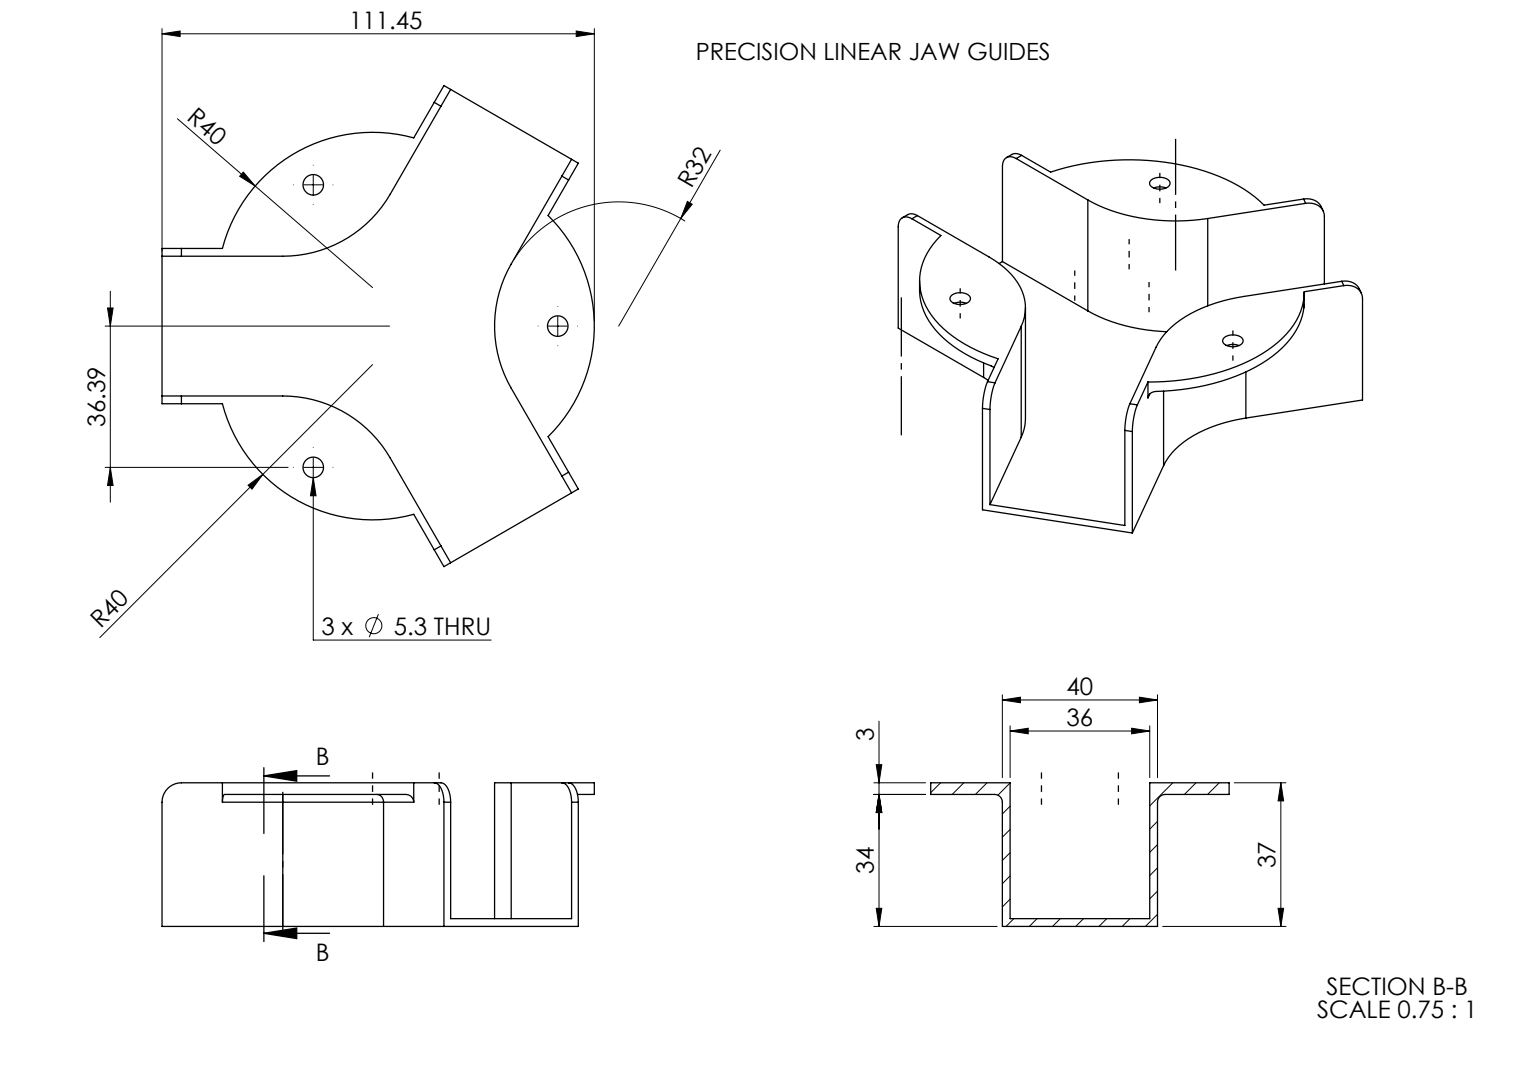
ISO-10303-21;
HEADER;
FILE_DESCRIPTION (('STEP AP214'),
    '1' );
FILE_NAME ('Precision Linear Jaw Guides.step',
    '2026-10-08T13:56:24',
    ( '' ),
    ( '' ),
    'SwSTEP 2.0',
    'SolidWorks 2026',
    '' );
FILE_SCHEMA (( 'AUTOMOTIVE_DESIGN' ));
ENDSEC;

DATA;
#1=ORIENTED_EDGE ( 'NONE', *, *, #6878, .F. ) ;
#24=ORIENTED_EDGE ( 'NONE', *, *, #9310, .F. ) ;
#44=CARTESIAN_POINT ( 'NONE',  ( 45.58845726811988897, -5.000000000000004441, 42.96152422706634155 ) ) ;
#63=EDGE_CURVE ( 'NONE', #10036, #14429, #10056, .T. ) ;
#65=CARTESIAN_POINT ( 'NONE',  ( 4.896370289181515290, -5.000000000000000000, 48.48076211353313170 ) ) ;
#73=FACE_OUTER_BOUND ( 'NONE', #11557, .T. ) ;
#75=ORIENTED_EDGE ( 'NONE', *, *, #13958, .T. ) ;
#102=EDGE_CURVE ( 'NONE', #3403, #4061, #7930, .T. ) ;
#103=CARTESIAN_POINT ( 'NONE',  ( 40.98096197216263903, -3.000000000000000000, 26.98110827883376928 ) ) ;
#118=DIRECTION ( 'NONE',  ( 0.000000000000000000, 0.000000000000000000, -1.000000000000000000 ) ) ;
#135=EDGE_LOOP ( 'NONE', ( #5012, #11685, #4576, #2768 ) ) ;
#159=ORIENTED_EDGE ( 'NONE', *, *, #7096, .F. ) ;
#161=CARTESIAN_POINT ( 'NONE',  ( 11.91154273188013768, 0.000000000000000000, -56.63139720814412925 ) ) ;
#162=AXIS2_PLACEMENT_3D ( 'NONE', #1282, #2402, #6227 ) ;
#178=PRESENTATION_STYLE_ASSIGNMENT (( #1292 ) ) ;
#181=ORIENTED_EDGE ( 'NONE', *, *, #2624, .T. ) ;
#183=EDGE_CURVE ( 'NONE', #10747, #715, #1391, .T. ) ;
#184=ORIENTED_EDGE ( 'NONE', *, *, #8002, .F. ) ;
#191=CARTESIAN_POINT ( 'NONE',  ( 39.53738644055469820, -5.000000000000000000, -28.48076211352550047 ) ) ;
#200=( NAMED_UNIT ( * ) SI_UNIT ( $, .STERADIAN. ) SOLID_ANGLE_UNIT ( ) );
#201=ORIENTED_EDGE ( 'NONE', *, *, #2412, .F. ) ;
#202=FACE_OUTER_BOUND ( 'NONE', #2206, .T. ) ;
#205=EDGE_CURVE ( 'NONE', #14772, #10685, #7688, .T. ) ;
#213=AXIS2_PLACEMENT_3D ( 'NONE', #6440, #11355, #304 ) ;
#233=VECTOR ( 'NONE', #8677, 1000.000000000000114 ) ;
#254=ORIENTED_EDGE ( 'NONE', *, *, #15050, .F. ) ;
#275=EDGE_CURVE ( 'NONE', #7055, #3403, #5959, .T. ) ;
#285=ORIENTED_EDGE ( 'NONE', *, *, #7627, .F. ) ;
#287=CARTESIAN_POINT ( 'NONE',  ( -28.86751345948129455, -35.00000000000000000, 49.99999999999999289 ) ) ;
#304=DIRECTION ( 'NONE',  ( 0.000000000000000000, 0.000000000000000000, 1.000000000000000000 ) ) ;
#342=FILL_AREA_STYLE ('',( #5011 ) ) ;
#347=AXIS2_PLACEMENT_3D ( 'NONE', #11601, #15335, #628 ) ;
#359=ORIENTED_EDGE ( 'NONE', *, *, #11812, .F. ) ;
#362=VERTEX_POINT ( 'NONE', #11512 ) ;
#381=ADVANCED_FACE ( 'NONE', ( #13861 ), #3996, .T. ) ;
#388=PLANE ( 'NONE',  #14679 ) ;
#395=VERTEX_POINT ( 'NONE', #15166 ) ;
#421=CARTESIAN_POINT ( 'NONE',  ( -44.05158835363087633, -3.098194602941751530, 21.36784885013319624 ) ) ;
#425=DIRECTION ( 'NONE',  ( -1.000000000000000000, 0.000000000000000000, 0.000000000000000000 ) ) ;
#435=LINE ( 'NONE', #9087, #7748 ) ;
#441=CIRCLE ( 'NONE', #4826, 29.99999999999999289 ) ;
#465=DIRECTION ( 'NONE',  ( 8.673617379884034486E-16, 0.000000000000000000, 1.000000000000000000 ) ) ;
#475=EDGE_CURVE ( 'NONE', #1675, #4627, #623, .T. ) ;
#478=EDGE_LOOP ( 'NONE', ( #2495, #13300, #2111, #13302 ) ) ;
#482=VERTEX_POINT ( 'NONE', #13120 ) ;
#487=ORIENTED_EDGE ( 'NONE', *, *, #7096, .T. ) ;
#492=AXIS2_PLACEMENT_3D ( 'NONE', #7401, #13083, #5207 ) ;
#512=VECTOR ( 'NONE', #11630, 1000.000000000000000 ) ;
#516=CARTESIAN_POINT ( 'NONE',  ( 47.32050807568879947, -37.00000000000000711, -41.96152422706630603 ) ) ;
#519=ADVANCED_FACE ( 'NONE', ( #932 ), #7080, .T. ) ;
#526=EDGE_LOOP ( 'NONE', ( #2721, #11527, #12496, #1351, #6317, #10390, #12512 ) ) ;
#534=EDGE_CURVE ( 'NONE', #9400, #9517, #9860, .T. ) ;
#536=DIRECTION ( 'NONE',  ( -0.8660254037844388186, -0.000000000000000000, 0.4999999999999998890 ) ) ;
#543=ORIENTED_EDGE ( 'NONE', *, *, #4679, .T. ) ;
#551=DIRECTION ( 'NONE',  ( -0.000000000000000000, 1.000000000000000000, -0.000000000000000000 ) ) ;
#560=VERTEX_POINT ( 'NONE', #14792 ) ;
#569=DIRECTION ( 'NONE',  ( -0.000000000000000000, -1.000000000000000000, -0.000000000000000000 ) ) ;
#575=CARTESIAN_POINT ( 'NONE',  ( 31.75426480542942898, -4.999999999999997335, -14.99999999999999645 ) ) ;
#581=CARTESIAN_POINT ( 'NONE',  ( -43.85680617780057844, -3.000000000000000000, 22.00000000000000355 ) ) ;
#585=EDGE_CURVE ( 'NONE', #1848, #15683, #12358, .T. ) ;
#593=AXIS2_PLACEMENT_3D ( 'NONE', #15441, #2156, #1919 ) ;
#600=EDGE_CURVE ( 'NONE', #4642, #13521, #7060, .T. ) ;
#612=CARTESIAN_POINT ( 'NONE',  ( 33.48631561299831105, -5.000000000000000000, -13.99999999999999645 ) ) ;
#621=VERTEX_POINT ( 'NONE', #4934 ) ;
#623=LINE ( 'NONE', #9571, #6285 ) ;
#626=DIRECTION ( 'NONE',  ( 0.5000000000000002220, -8.673617379884032514E-16, -0.8660254037844383745 ) ) ;
#628=DIRECTION ( 'NONE',  ( 0.000000000000000000, 0.000000000000000000, 1.000000000000000000 ) ) ;
#659=ORIENTED_EDGE ( 'NONE', *, *, #6025, .F. ) ;
#662=CARTESIAN_POINT ( 'NONE',  ( 21.91530404931195974, -5.000000000000000000, 6.041579923271729768 ) ) ;
#664=DIRECTION ( 'NONE',  ( 0.5000000000000001110, 0.000000000000000000, -0.8660254037844384856 ) ) ;
#682=CARTESIAN_POINT ( 'NONE',  ( 39.53738644056437579, -4.865128266864617856, 28.48076211354233322 ) ) ;
#690=LINE ( 'NONE', #4556, #8733 ) ;
#692=ORIENTED_EDGE ( 'NONE', *, *, #3560, .T. ) ;
#699=AXIS2_PLACEMENT_3D ( 'NONE', #5152, #6207, #10241 ) ;
#701=VECTOR ( 'NONE', #13836, 1000.000000000000000 ) ;
#702=CARTESIAN_POINT ( 'NONE',  ( 30.02221399786052913, -35.00000000000000000, 16.00000000000000000 ) ) ;
#703=TOROIDAL_SURFACE ( 'NONE', #4044, 28.00000000000000355, 2.000000000000000000 ) ;
#715=VERTEX_POINT ( 'NONE', #575 ) ;
#716=CARTESIAN_POINT ( 'NONE',  ( -60.00000000000000000, -4.999999999999997335, 19.99999999999999289 ) ) ;
#734=EDGE_CURVE ( 'NONE', #8265, #3643, #11314, .T. ) ;
#742=VERTEX_POINT ( 'NONE', #5180 ) ;
#743=CARTESIAN_POINT ( 'NONE',  ( -55.00000000000000000, -5.000000000000000000, -20.00000000000000711 ) ) ;
#754=CIRCLE ( 'NONE', #9773, 4.999999999999997335 ) ;
#762=EDGE_CURVE ( 'NONE', #10581, #8118, #3944, .T. ) ;
#764=DIRECTION ( 'NONE',  ( 0.000000000000000000, 0.000000000000000000, 1.000000000000000000 ) ) ;
#782=LINE ( 'NONE', #14580, #15415 ) ;
#784=CARTESIAN_POINT ( 'NONE',  ( -28.86751345948126257, 88.59290746114278647, -50.00000000000000711 ) ) ;
#786=PLANE ( 'NONE',  #13756 ) ;
#797=CARTESIAN_POINT ( 'NONE',  ( 31.75426480542940766, -37.00000000000000711, 15.00000000000001243 ) ) ;
#803=CARTESIAN_POINT ( 'NONE',  ( 4.095339645587086963, -3.395032785697071009, 48.69265741069611408 ) ) ;
#823=FACE_OUTER_BOUND ( 'NONE', #9623, .T. ) ;
#827=ORIENTED_EDGE ( 'NONE', *, *, #12141, .F. ) ;
#839=LINE ( 'NONE', #5761, #4644 ) ;
#840=CARTESIAN_POINT ( 'NONE',  ( 11.91154273188014301, -5.000000000000000000, -56.63139720814413636 ) ) ;
#850=AXIS2_PLACEMENT_3D ( 'NONE', #4119, #1694, #1775 ) ;
#855=DIRECTION ( 'NONE',  ( -0.8660254037844387076, -0.000000000000000000, -0.5000000000000003331 ) ) ;
#866=DIRECTION ( 'NONE',  ( 1.000000000000000000, -0.000000000000000000, 1.114413700119375779E-16 ) ) ;
#868=ORIENTED_EDGE ( 'NONE', *, *, #15692, .F. ) ;
#879=PLANE ( 'NONE',  #593 ) ;
#890=ORIENTED_EDGE ( 'NONE', *, *, #4257, .T. ) ;
#891=EDGE_LOOP ( 'NONE', ( #10651, #6417, #11764, #201 ) ) ;
#900=CARTESIAN_POINT ( 'NONE',  ( 40.53271815135278899, -3.097286126993895827, -27.46394321569970742 ) ) ;
#905=EDGE_CURVE ( 'NONE', #560, #1675, #15053, .T. ) ;
#923=CIRCLE ( 'NONE', #10224, 39.99999999999999289 ) ;
#925=EDGE_CURVE ( 'NONE', #3643, #15644, #11415, .T. ) ;
#932=FACE_OUTER_BOUND ( 'NONE', #10497, .T. ) ;
#947=CIRCLE ( 'NONE', #5073, 2.649999999999992806 ) ;
#954=CARTESIAN_POINT ( 'NONE',  ( -28.86751345948129455, -37.00000000000000711, 49.99999999999999289 ) ) ;
#978=CARTESIAN_POINT ( 'NONE',  ( 40.62171971187174790, -3.060691311048529872, -27.36941859593484949 ) ) ;
#984=CARTESIAN_POINT ( 'NONE',  ( 4.896370289182470081, -5.000000000000000000, -48.48076211353470910 ) ) ;
#991=EDGE_CURVE ( 'NONE', #3918, #7223, #6486, .T. ) ;
#999=ORIENTED_EDGE ( 'NONE', *, *, #10649, .T. ) ;
#1014=LINE ( 'NONE', #9427, #7731 ) ;
#1023=ORIENTED_EDGE ( 'NONE', *, *, #8305, .F. ) ;
#1039=ORIENTED_EDGE ( 'NONE', *, *, #7878, .T. ) ;
#1064=PLANE ( 'NONE',  #10813 ) ;
#1084=LINE ( 'NONE', #9647, #11321 ) ;
#1093=ORIENTED_EDGE ( 'NONE', *, *, #275, .T. ) ;
#1094=EDGE_CURVE ( 'NONE', #4540, #13587, #9387, .T. ) ;
#1101=CARTESIAN_POINT ( 'NONE',  ( -5.725490332117415093, -5.000000000000000000, 22.00000000000001421 ) ) ;
#1125=APPLICATION_CONTEXT ( 'automotive_design' ) ;
#1157=CIRCLE ( 'NONE', #15121, 2.000000000000000000 ) ;
#1168=DIRECTION ( 'NONE',  ( -0.4999999999999993894, 2.324088772396453021E-16, -0.8660254037844390407 ) ) ;
#1176=EDGE_CURVE ( 'NONE', #13609, #12316, #3175, .T. ) ;
#1183=AXIS2_PLACEMENT_3D ( 'NONE', #8469, #10583, #14590 ) ;
#1191=VECTOR ( 'NONE', #6258, 1000.000000000000114 ) ;
#1199=ORIENTED_EDGE ( 'NONE', *, *, #13990, .T. ) ;
#1228=ORIENTED_EDGE ( 'NONE', *, *, #10879, .T. ) ;
#1231=VECTOR ( 'NONE', #11987, 1000.000000000000000 ) ;
#1232=VERTEX_POINT ( 'NONE', #12353 ) ;
#1238=VECTOR ( 'NONE', #13025, 1000.000000000000000 ) ;
#1252=ORIENTED_EDGE ( 'NONE', *, *, #10295, .F. ) ;
#1278=EDGE_CURVE ( 'NONE', #482, #13637, #7445, .T. ) ;
#1282=CARTESIAN_POINT ( 'NONE',  ( 42.02221399786069611, -3.000000000000000000, 1.040834085586084257E-13 ) ) ;
#1292=SURFACE_STYLE_USAGE ( .BOTH. , #9862 ) ;
#1297=CARTESIAN_POINT ( 'NONE',  ( -5.725490332106780933, -3.000000000000000000, -9.916840153467775920 ) ) ;
#1301=CARTESIAN_POINT ( 'NONE',  ( 40.53089410526170866, -3.098194602941708009, 27.46587016624057753 ) ) ;
#1312=CARTESIAN_POINT ( 'NONE',  ( 31.75426480542942898, -37.00000000000000711, -14.99999999999999645 ) ) ;
#1317=CYLINDRICAL_SURFACE ( 'NONE', #10718, 2.649999999999992806 ) ;
#1321=LINE ( 'NONE', #13758, #7982 ) ;
#1327=ORIENTED_EDGE ( 'NONE', *, *, #11619, .T. ) ;
#1332=ORIENTED_EDGE ( 'NONE', *, *, #2188, .T. ) ;
#1336=DIRECTION ( 'NONE',  ( -0.000000000000000000, 1.000000000000000000, -0.000000000000000000 ) ) ;
#1345=ADVANCED_FACE ( 'NONE', ( #14048 ), #6389, .F. ) ;
#1349=LINE ( 'NONE', #2473, #9954 ) ;
#1351=ORIENTED_EDGE ( 'NONE', *, *, #2624, .F. ) ;
#1358=CARTESIAN_POINT ( 'NONE',  ( -60.00000000000000000, 88.59290746114278647, -18.00000000000001066 ) ) ;
#1370=ORIENTED_EDGE ( 'NONE', *, *, #10083, .T. ) ;
#1376=CIRCLE ( 'NONE', #12467, 5.000000000000001776 ) ;
#1378=EDGE_CURVE ( 'NONE', #15644, #3643, #6798, .T. ) ;
#1390=CARTESIAN_POINT ( 'NONE',  ( 45.58845726811992449, 88.59290746114278647, -42.96152422706630603 ) ) ;
#1391=LINE ( 'NONE', #1312, #701 ) ;
#1408=CARTESIAN_POINT ( 'NONE',  ( -28.86751345948129810, -3.000000000000000000, 22.00000000000000711 ) ) ;
#1436=DIRECTION ( 'NONE',  ( 0.8660254037844383745, 0.000000000000000000, 0.5000000000000004441 ) ) ;
#1437=ORIENTED_EDGE ( 'NONE', *, *, #6878, .T. ) ;
#1454=CIRCLE ( 'NONE', #10504, 4.999999999999997335 ) ;
#1461=AXIS2_PLACEMENT_3D ( 'NONE', #4140, #2767, #5035 ) ;
#1465=AXIS2_PLACEMENT_3D ( 'NONE', #3196, #3040, #12886 ) ;
#1474=CARTESIAN_POINT ( 'NONE',  ( 4.474605093962741975, -3.763931520638213346, -48.59453411586688532 ) ) ;
#1475=( LENGTH_UNIT ( ) NAMED_UNIT ( * ) SI_UNIT ( .MILLI., .METRE. ) );
#1479=DIRECTION ( 'NONE',  ( -0.000000000000000000, 1.000000000000000000, -0.000000000000000000 ) ) ;
#1501=PLANE ( 'NONE',  #213 ) ;
#1502=AXIS2_PLACEMENT_3D ( 'NONE', #3113, #6915, #14339 ) ;
#1503=LINE ( 'NONE', #9031, #12792 ) ;
#1509=ADVANCED_FACE ( 'NONE', ( #3066 ), #879, .F. ) ;
#1535=CARTESIAN_POINT ( 'NONE',  ( -44.37834814142158280, -4.097106062772742696, -20.21050050139519172 ) ) ;
#1536=CARTESIAN_POINT ( 'NONE',  ( 39.53738644056087992, 0.000000000000000000, -28.48076211352192999 ) ) ;
#1542=ORIENTED_EDGE ( 'NONE', *, *, #3362, .T. ) ;
#1556=ORIENTED_EDGE ( 'NONE', *, *, #13908, .T. ) ;
#1558=CARTESIAN_POINT ( 'NONE',  ( 4.623788282402106375, -3.982459619753664803, -48.55488344125860323 ) ) ;
#1559=VERTEX_POINT ( 'NONE', #8088 ) ;
#1571=EDGE_CURVE ( 'NONE', #10747, #11884, #6000, .T. ) ;
#1574=EDGE_CURVE ( 'NONE', #13609, #12993, #6074, .T. ) ;
#1575=ORIENTED_EDGE ( 'NONE', *, *, #762, .F. ) ;
#1600=CARTESIAN_POINT ( 'NONE',  ( -55.00000000000000000, 0.000000000000000000, -18.00000000000001066 ) ) ;
#1615=ORIENTED_EDGE ( 'NONE', *, *, #3613, .F. ) ;
#1619=LINE ( 'NONE', #5103, #7647 ) ;
#1622=EDGE_CURVE ( 'NONE', #10806, #15506, #12697, .T. ) ;
#1628=VECTOR ( 'NONE', #11144, 1000.000000000000000 ) ;
#1631=ORIENTED_EDGE ( 'NONE', *, *, #15956, .F. ) ;
#1634=CARTESIAN_POINT ( 'NONE',  ( -21.01110699893060030, -3.000000000000000000, 39.04230484541323420 ) ) ;
#1636=ORIENTED_EDGE ( 'NONE', *, *, #9965, .T. ) ;
#1638=FACE_OUTER_BOUND ( 'NONE', #14267, .T. ) ;
#1644=LINE ( 'NONE', #11268, #8249 ) ;
#1647=ORIENTED_EDGE ( 'NONE', *, *, #7708, .F. ) ;
#1648=DIRECTION ( 'NONE',  ( 0.000000000000000000, 1.000000000000000000, 0.000000000000000000 ) ) ;
#1661=FACE_OUTER_BOUND ( 'NONE', #5077, .T. ) ;
#1675=VERTEX_POINT ( 'NONE', #13291 ) ;
#1681=ADVANCED_FACE ( 'NONE', ( #12088 ), #2318, .F. ) ;
#1694=DIRECTION ( 'NONE',  ( -0.000000000000000000, -1.000000000000000000, -0.000000000000000000 ) ) ;
#1700=CARTESIAN_POINT ( 'NONE',  ( -44.32140357639302408, -3.763931520639085093, 20.42214537465778790 ) ) ;
#1708=CARTESIAN_POINT ( 'NONE',  ( 12.67949192431126093, -37.00000000000000711, -61.96152422706632024 ) ) ;
#1715=DIRECTION ( 'NONE',  ( -0.000000000000000000, -1.000000000000000000, -0.000000000000000000 ) ) ;
#1720=LINE ( 'NONE', #7962, #13361 ) ;
#1724=CARTESIAN_POINT ( 'NONE',  ( 43.08845726811987475, -5.000000000000000000, 38.63139720814412925 ) ) ;
#1740=ADVANCED_BREP_SHAPE_REPRESENTATION ( '', ( #14760, #3223 ), #14881 ) ;
#1745=DIRECTION ( 'NONE',  ( 0.000000000000000000, 0.000000000000000000, -1.000000000000000000 ) ) ;
#1746=DIRECTION ( 'NONE',  ( 0.4999999999999998335, 0.000000000000000000, 0.8660254037844387076 ) ) ;
#1748=CARTESIAN_POINT ( 'NONE',  ( 57.73502691896258199, -4.999999999999997335, 2.081668171172168513E-14 ) ) ;
#1754=AXIS2_PLACEMENT_3D ( 'NONE', #8234, #13131, #12807 ) ;
#1757=ORIENTED_EDGE ( 'NONE', *, *, #102, .T. ) ;
#1764=VERTEX_POINT ( 'NONE', #2950 ) ;
#1775=DIRECTION ( 'NONE',  ( 0.000000000000000000, 0.000000000000000000, -1.000000000000000000 ) ) ;
#1776=VECTOR ( 'NONE', #2352, 1000.000000000000227 ) ;
#1781=ORIENTED_EDGE ( 'NONE', *, *, #734, .T. ) ;
#1784=EDGE_LOOP ( 'NONE', ( #12318, #3642, #1, #11085, #9014 ) ) ;
#1785=LINE ( 'NONE', #3156, #7127 ) ;
#1805=DIRECTION ( 'NONE',  ( 0.5000000000000001110, 7.511572993685796142E-16, -0.8660254037844387076 ) ) ;
#1808=EDGE_LOOP ( 'NONE', ( #14146, #8988, #5187, #10193, #12157, #10854 ) ) ;
#1809=DIRECTION ( 'NONE',  ( -3.343241100358131282E-16, 0.000000000000000000, 1.000000000000000000 ) ) ;
#1810=DIRECTION ( 'NONE',  ( 3.343241100358131282E-16, -0.000000000000000000, -1.000000000000000000 ) ) ;
#1813=ORIENTED_EDGE ( 'NONE', *, *, #12598, .F. ) ;
#1822=CYLINDRICAL_SURFACE ( 'NONE', #11417, 39.99999999999999289 ) ;
#1823=LINE ( 'NONE', #8147, #2279 ) ;
#1832=EDGE_LOOP ( 'NONE', ( #10362, #15744, #11743, #14616, #184, #15244, #1199, #12170 ) ) ;
#1839=ADVANCED_FACE ( 'NONE', ( #1661 ), #3169, .F. ) ;
#1842=ADVANCED_FACE ( 'NONE', ( #6693 ), #12887, .F. ) ;
#1845=DIRECTION ( 'NONE',  ( -0.000000000000000000, 1.000000000000000000, -0.000000000000000000 ) ) ;
#1848=VERTEX_POINT ( 'NONE', #12962 ) ;
#1852=ORIENTED_EDGE ( 'NONE', *, *, #10275, .F. ) ;
#1857=FACE_OUTER_BOUND ( 'NONE', #10826, .T. ) ;
#1859=ADVANCED_FACE ( 'NONE', ( #14115 ), #10400, .T. ) ;
#1862=CARTESIAN_POINT ( 'NONE',  ( 42.02221399786069611, -3.000000000000001332, 2.650000000000089617 ) ) ;
#1869=ORIENTED_EDGE ( 'NONE', *, *, #7311, .F. ) ;
#1895=ADVANCED_FACE ( 'NONE', ( #9348 ), #1822, .T. ) ;
#1916=AXIS2_PLACEMENT_3D ( 'NONE', #14309, #3234, #12422 ) ;
#1919=DIRECTION ( 'NONE',  ( 0.4999999999999997224, 0.000000000000000000, 0.8660254037844388186 ) ) ;
#1930=EDGE_LOOP ( 'NONE', ( #5183, #3848, #7111, #15399 ) ) ;
#1941=VECTOR ( 'NONE', #5042, 1000.000000000000114 ) ;
#1950=EDGE_CURVE ( 'NONE', #11709, #1967, #4570, .T. ) ;
#1954=CIRCLE ( 'NONE', #9691, 40.00000000000000711 ) ;
#1967=VERTEX_POINT ( 'NONE', #4808 ) ;
#1986=FACE_OUTER_BOUND ( 'NONE', #5078, .T. ) ;
#1994=VERTEX_POINT ( 'NONE', #11032 ) ;
#2008=CARTESIAN_POINT ( 'NONE',  ( -21.01110699893060030, -3.000000000000000000, 36.39230484541324273 ) ) ;
#2009=VECTOR ( 'NONE', #13532, 1000.000000000000114 ) ;
#2047=DIRECTION ( 'NONE',  ( -0.5000000000000002220, 1.734723475976806503E-15, -0.8660254037844383745 ) ) ;
#2050=ORIENTED_EDGE ( 'NONE', *, *, #6025, .T. ) ;
#2063=CARTESIAN_POINT ( 'NONE',  ( -28.86751345948129455, -4.999999999999997335, 49.99999999999999289 ) ) ;
#2079=EDGE_CURVE ( 'NONE', #7857, #3918, #14581, .T. ) ;
#2087=DIRECTION ( 'NONE',  ( 0.000000000000000000, 0.000000000000000000, 1.000000000000000000 ) ) ;
#2094=DIRECTION ( 'NONE',  ( 0.000000000000000000, -1.000000000000000000, 0.000000000000000000 ) ) ;
#2105=DIRECTION ( 'NONE',  ( 0.8660254037844388186, 0.000000000000000000, -0.4999999999999996669 ) ) ;
#2107=DIRECTION ( 'NONE',  ( 0.5000000000000002220, -0.000000000000000000, -0.8660254037844384856 ) ) ;
#2111=ORIENTED_EDGE ( 'NONE', *, *, #14976, .F. ) ;
#2121=VERTEX_POINT ( 'NONE', #1708 ) ;
#2147=EDGE_LOOP ( 'NONE', ( #8319, #4838, #7537, #3603 ) ) ;
#2156=DIRECTION ( 'NONE',  ( -0.8660254037844388186, 0.000000000000000000, 0.4999999999999997224 ) ) ;
#2159=DIRECTION ( 'NONE',  ( 0.000000000000000000, 1.000000000000000000, 0.000000000000000000 ) ) ;
#2176=CARTESIAN_POINT ( 'NONE',  ( 39.73946572741719052, -3.978804951770217091, -28.28016224734468409 ) ) ;
#2179=DIRECTION ( 'NONE',  ( -0.5000000000000002220, 0.000000000000000000, 0.8660254037844384856 ) ) ;
#2184=ORIENTED_EDGE ( 'NONE', *, *, #11259, .T. ) ;
#2188=EDGE_CURVE ( 'NONE', #15092, #15644, #6807, .T. ) ;
#2193=CARTESIAN_POINT ( 'NONE',  ( 40.11295108777448348, -3.387975324183181591, 27.90213124783379328 ) ) ;
#2206=EDGE_LOOP ( 'NONE', ( #7820, #14661, #10147, #6463, #13439 ) ) ;
#2228=DIRECTION ( 'NONE',  ( 0.4999999999999997224, 0.000000000000000000, 0.8660254037844387076 ) ) ;
#2232=CARTESIAN_POINT ( 'NONE',  ( 4.472333508125966972, -3.761076017575723629, 48.59513319789044772 ) ) ;
#2243=VERTEX_POINT ( 'NONE', #15539 ) ;
#2245=EDGE_LOOP ( 'NONE', ( #692, #3137, #868, #3826 ) ) ;
#2252=AXIS2_PLACEMENT_3D ( 'NONE', #12708, #1648, #5213 ) ;
#2253=FACE_OUTER_BOUND ( 'NONE', #9899, .T. ) ;
#2272=AXIS2_PLACEMENT_3D ( 'NONE', #3749, #8697, #7653 ) ;
#2276=FACE_BOUND ( 'NONE', #7389, .T. ) ;
#2279=VECTOR ( 'NONE', #1746, 1000.000000000000114 ) ;
#2286=EDGE_LOOP ( 'NONE', ( #1437, #8006, #10768, #7115, #2904, #11120, #4080, #10979 ) ) ;
#2290=ORIENTED_EDGE ( 'NONE', *, *, #12191, .F. ) ;
#2291=CYLINDRICAL_SURFACE ( 'NONE', #7229, 30.00000000000000711 ) ;
#2297=LINE ( 'NONE', #3424, #6588 ) ;
#2309=CARTESIAN_POINT ( 'NONE',  ( -43.85680617780057844, -3.000000000000000000, 22.00000000000000355 ) ) ;
#2316=EDGE_CURVE ( 'NONE', #2243, #9104, #9389, .T. ) ;
#2318=CYLINDRICAL_SURFACE ( 'NONE', #10138, 2.000000000000001776 ) ;
#2340=CARTESIAN_POINT ( 'NONE',  ( 0.000000000000000000, 0.000000000000000000, 0.000000000000000000 ) ) ;
#2344=DIRECTION ( 'NONE',  ( 0.000000000000000000, -0.000000000000000000, -1.000000000000000000 ) ) ;
#2352=DIRECTION ( 'NONE',  ( 0.5000000000000001110, 0.000000000000000000, -0.8660254037844384856 ) ) ;
#2362=ORIENTED_EDGE ( 'NONE', *, *, #15794, .F. ) ;
#2365=EDGE_CURVE ( 'NONE', #9517, #7038, #8277, .T. ) ;
#2379=VERTEX_POINT ( 'NONE', #14713 ) ;
#2384=ADVANCED_FACE ( 'NONE', ( #13402, #3636 ), #2654, .T. ) ;
#2387=DIRECTION ( 'NONE',  ( -3.343241100358131282E-16, -0.000000000000000000, 1.000000000000000000 ) ) ;
#2398=DIRECTION ( 'NONE',  ( -0.000000000000000000, 1.000000000000000000, -0.000000000000000000 ) ) ;
#2402=DIRECTION ( 'NONE',  ( -0.000000000000000000, -1.000000000000000000, -0.000000000000000000 ) ) ;
#2412=EDGE_CURVE ( 'NONE', #12993, #5955, #6064, .T. ) ;
#2416=ORIENTED_EDGE ( 'NONE', *, *, #8575, .F. ) ;
#2430=CARTESIAN_POINT ( 'NONE',  ( 43.08845726811992449, 0.000000000000000000, -38.63139720814411504 ) ) ;
#2453=CARTESIAN_POINT ( 'NONE',  ( 31.75426480542940766, -37.00000000000000711, 15.00000000000001066 ) ) ;
#2457=VERTEX_POINT ( 'NONE', #6311 ) ;
#2473=CARTESIAN_POINT ( 'NONE',  ( 45.58845726811988897, -5.000000000000000000, 42.96152422706632734 ) ) ;
#2476=CARTESIAN_POINT ( 'NONE',  ( 12.67949192431120586, -37.00000000000000711, 61.96152422706632024 ) ) ;
#2478=CARTESIAN_POINT ( 'NONE',  ( -16.18981371719799611, -5.000000000000000000, -15.95842007673748952 ) ) ;
#2479=VERTEX_POINT ( 'NONE', #4929 ) ;
#2480=CARTESIAN_POINT ( 'NONE',  ( 40.98096197216263903, -3.000000000000000000, 26.98110827883376928 ) ) ;
#2495=ORIENTED_EDGE ( 'NONE', *, *, #11437, .T. ) ;
#2511=CARTESIAN_POINT ( 'NONE',  ( 4.830276029870151255, -4.472255266397859863, -48.49891554519376058 ) ) ;
#2519=CARTESIAN_POINT ( 'NONE',  ( 45.58845726811992449, 0.000000000000000000, -42.96152422706630603 ) ) ;
#2531=DIRECTION ( 'NONE',  ( 0.000000000000000000, 1.000000000000000000, 0.000000000000000000 ) ) ;
#2538=ORIENTED_EDGE ( 'NONE', *, *, #14897, .F. ) ;
#2547=EDGE_CURVE ( 'NONE', #13637, #6536, #8775, .T. ) ;
#2558=ORIENTED_EDGE ( 'NONE', *, *, #4185, .T. ) ;
#2565=ORIENTED_EDGE ( 'NONE', *, *, #13620, .T. ) ;
#2600=EDGE_LOOP ( 'NONE', ( #15728, #10436, #7534, #8946 ) ) ;
#2601=LINE ( 'NONE', #7553, #12108 ) ;
#2610=PLANE ( 'NONE',  #11285 ) ;
#2619=CARTESIAN_POINT ( 'NONE',  ( -21.01110699893041911, -3.000000000000001332, -33.74230484541335784 ) ) ;
#2624=EDGE_CURVE ( 'NONE', #7223, #8388, #4671, .T. ) ;
#2628=CARTESIAN_POINT ( 'NONE',  ( -5.725490332117410652, -3.000000000000000000, 49.91684015347181003 ) ) ;
#2642=ORIENTED_EDGE ( 'NONE', *, *, #7627, .T. ) ;
#2643=ADVANCED_FACE ( 'NONE', ( #6871 ), #12910, .F. ) ;
#2654=PLANE ( 'NONE',  #3400 ) ;
#2660=SURFACE_STYLE_FILL_AREA ( #342 ) ;
#2663=ADVANCED_FACE ( 'NONE', ( #14379, #8092 ), #12010, .T. ) ;
#2665=ORIENTED_EDGE ( 'NONE', *, *, #3366, .T. ) ;
#2704=ORIENTED_EDGE ( 'NONE', *, *, #13922, .T. ) ;
#2705=DIRECTION ( 'NONE',  ( 0.000000000000000000, 1.000000000000000000, 0.000000000000000000 ) ) ;
#2709=EDGE_CURVE ( 'NONE', #10113, #15266, #15594, .T. ) ;
#2719=AXIS2_PLACEMENT_3D ( 'NONE', #15918, #11211, #9916 ) ;
#2720=CARTESIAN_POINT ( 'NONE',  ( -60.00000000000000000, -4.999999999999997335, -20.00000000000000711 ) ) ;
#2721=ORIENTED_EDGE ( 'NONE', *, *, #7757, .T. ) ;
#2722=ORIENTED_EDGE ( 'NONE', *, *, #14976, .T. ) ;
#2737=CARTESIAN_POINT ( 'NONE',  ( -44.29779928441806902, -3.660959011663034612, -20.50864992044095558 ) ) ;
#2742=CARTESIAN_POINT ( 'NONE',  ( -1.154700538379255903, -35.00000000000000000, 34.00000000000000711 ) ) ;
#2748=CARTESIAN_POINT ( 'NONE',  ( -60.00000000000000000, -37.00000000000000711, -20.00000000000000711 ) ) ;
#2749=ORIENTED_EDGE ( 'NONE', *, *, #9020, .T. ) ;
#2751=CARTESIAN_POINT ( 'NONE',  ( -55.00000000000000000, -5.000000000000000000, 0.000000000000000000 ) ) ;
#2763=CARTESIAN_POINT ( 'NONE',  ( 4.686969894964994943, -4.098233149437105816, -48.53786474802608097 ) ) ;
#2764=ORIENTED_EDGE ( 'NONE', *, *, #15493, .F. ) ;
#2767=DIRECTION ( 'NONE',  ( 0.000000000000000000, 1.000000000000000000, 0.000000000000000000 ) ) ;
#2768=ORIENTED_EDGE ( 'NONE', *, *, #905, .F. ) ;
#2787=FACE_OUTER_BOUND ( 'NONE', #2245, .T. ) ;
#2791=DIRECTION ( 'NONE',  ( 0.000000000000000000, 0.000000000000000000, -1.000000000000000000 ) ) ;
#2809=CARTESIAN_POINT ( 'NONE',  ( -55.00000000000000000, 0.000000000000000000, 17.99999999999999289 ) ) ;
#2822=CARTESIAN_POINT ( 'NONE',  ( -44.43375672972994295, -5.000000000000000000, -20.00000000000000355 ) ) ;
#2862=EDGE_LOOP ( 'NONE', ( #1575, #5938 ) ) ;
#2870=CARTESIAN_POINT ( 'NONE',  ( 42.02221399786069611, 0.000000000000000000, 1.040834085586084257E-13 ) ) ;
#2871=DIRECTION ( 'NONE',  ( -0.000000000000000000, -1.000000000000000000, -0.000000000000000000 ) ) ;
#2888=ORIENTED_EDGE ( 'NONE', *, *, #10649, .F. ) ;
#2904=ORIENTED_EDGE ( 'NONE', *, *, #15532, .F. ) ;
#2914=VECTOR ( 'NONE', #3639, 1000.000000000000000 ) ;
#2934=EDGE_LOOP ( 'NONE', ( #12396, #10392, #8390, #1023 ) ) ;
#2942=VECTOR ( 'NONE', #7108, 1000.000000000000000 ) ;
#2944=CARTESIAN_POINT ( 'NONE',  ( -55.00000000000000000, -5.000000000000000000, 0.000000000000000000 ) ) ;
#2950=CARTESIAN_POINT ( 'NONE',  ( -21.01110699893060030, -3.000000000000001332, 39.04230484541322710 ) ) ;
#2953=DIRECTION ( 'NONE',  ( 0.8660254037844383745, -0.000000000000000000, 0.5000000000000004441 ) ) ;
#2961=ORIENTED_EDGE ( 'NONE', *, *, #600, .F. ) ;
#2967=DIRECTION ( 'NONE',  ( 0.000000000000000000, -1.000000000000000000, 0.000000000000000000 ) ) ;
#2983=CIRCLE ( 'NONE', #7129, 4.999999999999997335 ) ;
#2988=DIRECTION ( 'NONE',  ( 0.000000000000000000, -1.000000000000000000, 0.000000000000000000 ) ) ;
#2991=CIRCLE ( 'NONE', #6612, 2.649999999999985700 ) ;
#2994=AXIS2_PLACEMENT_3D ( 'NONE', #11453, #13957, #3785 ) ;
#3022=CARTESIAN_POINT ( 'NONE',  ( -60.00000000000000000, -37.00000000000000711, 19.99999999999999289 ) ) ;
#3029=ORIENTED_EDGE ( 'NONE', *, *, #925, .T. ) ;
#3031=AXIS2_PLACEMENT_3D ( 'NONE', #2944, #2791, #11360 ) ;
#3040=DIRECTION ( 'NONE',  ( -0.000000000000000000, 1.000000000000000000, -0.000000000000000000 ) ) ;
#3046=DIRECTION ( 'NONE',  ( 0.5000000000000002220, 0.000000000000000000, -0.8660254037844383745 ) ) ;
#3051=ORIENTED_EDGE ( 'NONE', *, *, #1378, .F. ) ;
#3064=CARTESIAN_POINT ( 'NONE',  ( 14.41154273188008439, -5.000000000000004441, 60.96152422706632024 ) ) ;
#3066=FACE_OUTER_BOUND ( 'NONE', #14680, .T. ) ;
#3078=ORIENTED_EDGE ( 'NONE', *, *, #9985, .F. ) ;
#3083=CARTESIAN_POINT ( 'NONE',  ( -43.93709122729256222, -3.012258285427890758, 21.74438836017856147 ) ) ;
#3099=EDGE_LOOP ( 'NONE', ( #3078, #14226, #5732, #14176, #2642 ) ) ;
#3107=DIRECTION ( 'NONE',  ( 0.000000000000000000, -1.000000000000000000, 0.000000000000000000 ) ) ;
#3113=CARTESIAN_POINT ( 'NONE',  ( -28.86751345948129455, -4.999999999999997335, 22.00000000000000711 ) ) ;
#3137=ORIENTED_EDGE ( 'NONE', *, *, #10177, .F. ) ;
#3147=LINE ( 'NONE', #10598, #6660 ) ;
#3156=CARTESIAN_POINT ( 'NONE',  ( 43.08845726811992449, 0.000000000000000000, -38.63139720814411504 ) ) ;
#3159=CARTESIAN_POINT ( 'NONE',  ( 40.98096197215471648, -3.000000000000000000, -26.98110827881998119 ) ) ;
#3162=EDGE_CURVE ( 'NONE', #12752, #4331, #6296, .T. ) ;
#3163=CARTESIAN_POINT ( 'NONE',  ( -55.00000000000000000, -5.000000000000000000, -18.00000000000001066 ) ) ;
#3169=TOROIDAL_SURFACE ( 'NONE', #5505, 27.99999999999998934, 2.000000000000000000 ) ;
#3175=CIRCLE ( 'NONE', #12189, 39.99999999999999289 ) ;
#3178=CARTESIAN_POINT ( 'NONE',  ( -28.86751345948126612, -35.00000000000000000, -18.00000000000000355 ) ) ;
#3187=CARTESIAN_POINT ( 'NONE',  ( -28.86751345948130165, 88.59290746114278647, 18.00000000000000355 ) ) ;
#3188=CARTESIAN_POINT ( 'NONE',  ( -55.00000000000000000, -5.000000000000000000, 17.99999999999999289 ) ) ;
#3189=ORIENTED_EDGE ( 'NONE', *, *, #585, .F. ) ;
#3193=DIRECTION ( 'NONE',  ( 0.4999999999999997224, 0.000000000000000000, 0.8660254037844387076 ) ) ;
#3196=CARTESIAN_POINT ( 'NONE',  ( -28.86751345948129455, -4.999999999999997335, 49.99999999999999289 ) ) ;
#3197=DIRECTION ( 'NONE',  ( -0.000000000000000000, 1.000000000000000000, -0.000000000000000000 ) ) ;
#3199=CARTESIAN_POINT ( 'NONE',  ( -2.886751345948139758, -37.00000000000000711, 35.00000000000000000 ) ) ;
#3206=CARTESIAN_POINT ( 'NONE',  ( -60.00000000000000000, 0.000000000000000000, -20.00000000000000711 ) ) ;
#3208=ORIENTED_EDGE ( 'NONE', *, *, #15815, .F. ) ;
#3214=AXIS2_PLACEMENT_3D ( 'NONE', #3999, #15168, #8711 ) ;
#3215=CARTESIAN_POINT ( 'NONE',  ( -44.43375672974056556, -5.000000000000000000, 20.00000000000000000 ) ) ;
#3223=AXIS2_PLACEMENT_3D ( 'NONE', #11897, #11972, #4638 ) ;
#3225=VECTOR ( 'NONE', #8211, 1000.000000000000000 ) ;
#3232=CARTESIAN_POINT ( 'NONE',  ( -5.725490332106780933, 0.000000000000000000, -9.916840153467775920 ) ) ;
#3234=DIRECTION ( 'NONE',  ( -0.000000000000000000, 1.000000000000000000, -0.000000000000000000 ) ) ;
#3236=ADVANCED_FACE ( 'NONE', ( #1986 ), #786, .F. ) ;
#3259=AXIS2_PLACEMENT_3D ( 'NONE', #3682, #4583, #2228 ) ;
#3262=CARTESIAN_POINT ( 'NONE',  ( -21.01110699893041911, -3.000000000000001332, -39.04230484541332657 ) ) ;
#3264=DIRECTION ( 'NONE',  ( 1.000000000000000000, -0.000000000000000000, 1.114413700119375779E-16 ) ) ;
#3298=EDGE_CURVE ( 'NONE', #1232, #12621, #8311, .T. ) ;
#3307=EDGE_CURVE ( 'NONE', #11884, #2379, #14118, .T. ) ;
#3362=EDGE_CURVE ( 'NONE', #14429, #395, #15202, .T. ) ;
#3366=EDGE_CURVE ( 'NONE', #362, #1764, #13893, .T. ) ;
#3379=CARTESIAN_POINT ( 'NONE',  ( 39.53738644056087992, -3.000000000000000000, -28.48076211352192999 ) ) ;
#3382=EDGE_CURVE ( 'NONE', #5667, #6319, #9012, .T. ) ;
#3385=ORIENTED_EDGE ( 'NONE', *, *, #585, .T. ) ;
#3387=VERTEX_POINT ( 'NONE', #4892 ) ;
#3394=CARTESIAN_POINT ( 'NONE',  ( 40.79999760747214310, -3.012271619929379973, -27.17815842419070194 ) ) ;
#3400=AXIS2_PLACEMENT_3D ( 'NONE', #2340, #5091, #14962 ) ;
#3403=VERTEX_POINT ( 'NONE', #6194 ) ;
#3415=DIRECTION ( 'NONE',  ( -1.000000000000000000, 0.000000000000000000, -3.343241100358131282E-16 ) ) ;
#3424=CARTESIAN_POINT ( 'NONE',  ( -60.00000000000000000, -37.00000000000000711, -20.00000000000000711 ) ) ;
#3441=LINE ( 'NONE', #8394, #9959 ) ;
#3444=AXIS2_PLACEMENT_3D ( 'NONE', #612, #1805, #5612 ) ;
#3445=EDGE_CURVE ( 'NONE', #6536, #9071, #1644, .T. ) ;
#3450=DIRECTION ( 'NONE',  ( 0.000000000000000000, -0.000000000000000000, 1.000000000000000000 ) ) ;
#3470=CARTESIAN_POINT ( 'NONE',  ( -21.01110699893041911, 0.000000000000000000, -39.04230484541333368 ) ) ;
#3485=CIRCLE ( 'NONE', #9438, 40.00000000000001421 ) ;
#3502=DIRECTION ( 'NONE',  ( 0.5000000000000005551, 0.000000000000000000, -0.8660254037844382635 ) ) ;
#3507=CARTESIAN_POINT ( 'NONE',  ( -4.618802153516977427, -3.000000000000000000, -36.00000000000000711 ) ) ;
#3511=DIRECTION ( 'NONE',  ( -0.000000000000000000, -1.000000000000000000, -0.000000000000000000 ) ) ;
#3559=EDGE_CURVE ( 'NONE', #6711, #2479, #1376, .T. ) ;
#3560=EDGE_CURVE ( 'NONE', #715, #7857, #10432, .T. ) ;
#3565=DIRECTION ( 'NONE',  ( -0.000000000000000000, 1.000000000000000000, -0.000000000000000000 ) ) ;
#3566=AXIS2_PLACEMENT_3D ( 'NONE', #840, #10853, #11969 ) ;
#3570=CARTESIAN_POINT ( 'NONE',  ( 39.73786839672636262, -3.982459619754358027, 28.28175983491992440 ) ) ;
#3572=AXIS2_PLACEMENT_3D ( 'NONE', #15699, #10763, #2105 ) ;
#3581=EDGE_CURVE ( 'NONE', #11709, #621, #11584, .T. ) ;
#3588=ORIENTED_EDGE ( 'NONE', *, *, #13516, .T. ) ;
#3597=DIRECTION ( 'NONE',  ( -0.000000000000000000, 1.000000000000000000, -0.000000000000000000 ) ) ;
#3603=ORIENTED_EDGE ( 'NONE', *, *, #11316, .F. ) ;
#3613=EDGE_CURVE ( 'NONE', #12316, #14284, #839, .T. ) ;
#3619=B_SPLINE_CURVE_WITH_KNOTS ( 'NONE', 3,
 ( #12756, #3961, #8911, #13812, #5259, #7704, #6558, #1700, #7786, #4040, #11473, #421, #5347, #3083, #9229, #581 ),
 .UNSPECIFIED., .F., .F.,
 ( 4, 2, 2, 2, 2, 2, 2, 4 ),
 ( 8.673617379884034509E-19, 0.0003988053453839040001, 0.0007976106907678071328, 0.001196416036151710157, 0.001595221381535612314, 0.002392832072303412074, 0.002791637417687314882, 0.003190442763071217255 ),
 .UNSPECIFIED. ) ;
#3624=ORIENTED_EDGE ( 'NONE', *, *, #3631, .F. ) ;
#3627=FACE_OUTER_BOUND ( 'NONE', #11745, .T. ) ;
#3631=EDGE_CURVE ( 'NONE', #15683, #15871, #5453, .T. ) ;
#3636=FACE_OUTER_BOUND ( 'NONE', #4460, .T. ) ;
#3639=DIRECTION ( 'NONE',  ( 0.000000000000000000, 0.000000000000000000, -1.000000000000000000 ) ) ;
#3642=ORIENTED_EDGE ( 'NONE', *, *, #9463, .T. ) ;
#3643=VERTEX_POINT ( 'NONE', #3262 ) ;
#3656=LINE ( 'NONE', #11098, #13351 ) ;
#3671=CARTESIAN_POINT ( 'NONE',  ( -21.01110699893060030, 0.000000000000000000, 36.39230484541324273 ) ) ;
#3675=AXIS2_PLACEMENT_3D ( 'NONE', #11479, #12607, #6561 ) ;
#3682=CARTESIAN_POINT ( 'NONE',  ( 27.49999999999998224, -5.000000000000000000, 47.63139720814412925 ) ) ;
#3691=CARTESIAN_POINT ( 'NONE',  ( -1.154700538379255903, 88.59290746114278647, 34.00000000000000711 ) ) ;
#3725=CIRCLE ( 'NONE', #7103, 2.649999999999985700 ) ;
#3730=DIRECTION ( 'NONE',  ( -0.4999999999999997224, 0.000000000000000000, -0.8660254037844388186 ) ) ;
#3739=ORIENTED_EDGE ( 'NONE', *, *, #8722, .F. ) ;
#3742=LINE ( 'NONE', #2519, #1941 ) ;
#3748=DIRECTION ( 'NONE',  ( -0.000000000000000000, -1.000000000000000000, -0.000000000000000000 ) ) ;
#3749=CARTESIAN_POINT ( 'NONE',  ( -5.725490332106780933, -3.000000000000000000, -9.916840153467775920 ) ) ;
#3751=ORIENTED_EDGE ( 'NONE', *, *, #3382, .T. ) ;
#3783=EDGE_CURVE ( 'NONE', #6940, #1967, #11009, .T. ) ;
#3785=DIRECTION ( 'NONE',  ( 0.000000000000000000, 0.000000000000000000, -1.000000000000000000 ) ) ;
#3801=( NAMED_UNIT ( * ) PLANE_ANGLE_UNIT ( ) SI_UNIT ( $, .RADIAN. ) );
#3819=CARTESIAN_POINT ( 'NONE',  ( 3.137352903976079244, -3.012258285427876547, -48.92283135131768290 ) ) ;
#3820=AXIS2_PLACEMENT_3D ( 'NONE', #10472, #10010, #9105 ) ;
#3826=ORIENTED_EDGE ( 'NONE', *, *, #5340, .F. ) ;
#3848=ORIENTED_EDGE ( 'NONE', *, *, #1278, .F. ) ;
#3871=VECTOR ( 'NONE', #10384, 1000.000000000000114 ) ;
#3886=FACE_OUTER_BOUND ( 'NONE', #14080, .T. ) ;
#3907=FACE_OUTER_BOUND ( 'NONE', #2286, .T. ) ;
#3915=FACE_BOUND ( 'NONE', #5233, .T. ) ;
#3918=VERTEX_POINT ( 'NONE', #10209 ) ;
#3944=CIRCLE ( 'NONE', #850, 2.649999999999985700 ) ;
#3946=AXIS2_PLACEMENT_3D ( 'NONE', #9061, #569, #12588 ) ;
#3952=CARTESIAN_POINT ( 'NONE',  ( -43.93697442715794210, -3.012271619929379085, -21.74475519031983950 ) ) ;
#3961=CARTESIAN_POINT ( 'NONE',  ( -44.43375672974056556, -4.865128266864608975, 19.99999999999999645 ) ) ;
#3982=CARTESIAN_POINT ( 'NONE',  ( 4.896370289192182312, -5.000000000000000000, -48.48076211352908871 ) ) ;
#3987=LINE ( 'NONE', #7486, #8753 ) ;
#3990=CARTESIAN_POINT ( 'NONE',  ( -2.886751345948103342, -37.00000000000000711, -35.00000000000000000 ) ) ;
#3996=CYLINDRICAL_SURFACE ( 'NONE', #3031, 4.999999999999997335 ) ;
#3999=CARTESIAN_POINT ( 'NONE',  ( 47.32050807568875683, -37.00000000000000711, 41.96152422706633445 ) ) ;
#4020=CARTESIAN_POINT ( 'NONE',  ( 4.896370289181002811, 0.000000000000000000, -48.48076211353215825 ) ) ;
#4039=ORIENTED_EDGE ( 'NONE', *, *, #3162, .T. ) ;
#4040=CARTESIAN_POINT ( 'NONE',  ( -44.22043002422942948, -3.387975324183347237, 20.78776903885821881 ) ) ;
#4044=AXIS2_PLACEMENT_3D ( 'NONE', #15755, #9591, #15826 ) ;
#4045=DIRECTION ( 'NONE',  ( -0.000000000000000000, -1.000000000000000000, -0.000000000000000000 ) ) ;
#4055=ORIENTED_EDGE ( 'NONE', *, *, #7862, .T. ) ;
#4056=CARTESIAN_POINT ( 'NONE',  ( 3.882512440569886980, -3.242827243955292094, -48.74656899134319588 ) ) ;
#4061=VERTEX_POINT ( 'NONE', #15002 ) ;
#4067=VECTOR ( 'NONE', #14769, 1000.000000000000114 ) ;
#4069=ADVANCED_FACE ( 'NONE', ( #3915, #9101 ), #1501, .F. ) ;
#4074=ORIENTED_EDGE ( 'NONE', *, *, #10083, .F. ) ;
#4075=CARTESIAN_POINT ( 'NONE',  ( -2.886751345948139758, -4.999999999999997335, 35.00000000000000000 ) ) ;
#4078=CARTESIAN_POINT ( 'NONE',  ( -5.725490332117410652, -3.000000000000000000, 9.916840153471811803 ) ) ;
#4080=ORIENTED_EDGE ( 'NONE', *, *, #14643, .T. ) ;
#4091=DIRECTION ( 'NONE',  ( -0.8660254037844383745, 0.000000000000000000, -0.5000000000000006661 ) ) ;
#4096=CARTESIAN_POINT ( 'NONE',  ( 12.67949192431120586, -4.999999999999997335, 61.96152422706632024 ) ) ;
#4116=CARTESIAN_POINT ( 'NONE',  ( -44.12168325659714441, -3.194220869028276066, -21.13058177393697434 ) ) ;
#4119=CARTESIAN_POINT ( 'NONE',  ( 42.02221399786069611, -3.000000000000001332, 1.040834085586084257E-13 ) ) ;
#4137=SURFACE_STYLE_USAGE ( .BOTH. , #13991 ) ;
#4140=CARTESIAN_POINT ( 'NONE',  ( -28.86751345948129455, 0.000000000000000000, 49.99999999999999289 ) ) ;
#4151=CARTESIAN_POINT ( 'NONE',  ( -60.00000000000000000, 88.59290746114278647, -18.00000000000001066 ) ) ;
#4168=CARTESIAN_POINT ( 'NONE',  ( 14.41154273188013590, -5.000000000000000000, -60.96152422706632024 ) ) ;
#4172=VECTOR ( 'NONE', #2179, 1000.000000000000000 ) ;
#4182=ORIENTED_EDGE ( 'NONE', *, *, #11259, .F. ) ;
#4185=EDGE_CURVE ( 'NONE', #12880, #15286, #1454, .T. ) ;
#4198=EDGE_CURVE ( 'NONE', #15286, #10806, #9264, .T. ) ;
#4202=CARTESIAN_POINT ( 'NONE',  ( -28.86751345948126612, 88.59290746114278647, -18.00000000000000355 ) ) ;
#4238=ORIENTED_EDGE ( 'NONE', *, *, #5340, .T. ) ;
#4253=EDGE_CURVE ( 'NONE', #2121, #1994, #11052, .T. ) ;
#4254=CARTESIAN_POINT ( 'NONE',  ( 27.50000000000003197, -5.000000000000000000, -47.63139720814412925 ) ) ;
#4257=EDGE_CURVE ( 'NONE', #5955, #4331, #5854, .T. ) ;
#4278=CARTESIAN_POINT ( 'NONE',  ( -43.85680617778868395, -3.000000000000000000, -22.00000000000000355 ) ) ;
#4301=SHAPE_DEFINITION_REPRESENTATION ( #8246, #6981 ) ;
#4304=EDGE_LOOP ( 'NONE', ( #12767, #3208, #12532, #11298 ) ) ;
#4308=ORIENTED_EDGE ( 'NONE', *, *, #6079, .F. ) ;
#4313=EDGE_CURVE ( 'NONE', #5426, #11703, #441, .T. ) ;
#4315=AXIS2_PLACEMENT_3D ( 'NONE', #2751, #11475, #425 ) ;
#4316=CARTESIAN_POINT ( 'NONE',  ( 11.45098066423670247, -3.000000000000000000, 1.122567565269603304E-11 ) ) ;
#4320=AXIS2_PLACEMENT_3D ( 'NONE', #15738, #13357, #7315 ) ;
#4331=VERTEX_POINT ( 'NONE', #7188 ) ;
#4336=ADVANCED_FACE ( 'NONE', ( #6125 ), #703, .F. ) ;
#4347=VERTEX_POINT ( 'NONE', #4829 ) ;
#4370=ORIENTED_EDGE ( 'NONE', *, *, #4253, .T. ) ;
#4377=CARTESIAN_POINT ( 'NONE',  ( -60.00000000000000000, -5.000000000000004441, -18.00000000000001066 ) ) ;
#4382=CARTESIAN_POINT ( 'NONE',  ( 39.57820647634153488, -4.462727778340672025, -28.44065064052909975 ) ) ;
#4400=CARTESIAN_POINT ( 'NONE',  ( 30.02221399786053624, -35.00000000000000000, -15.99999999999997868 ) ) ;
#4423=CYLINDRICAL_SURFACE ( 'NONE', #1183, 30.00000000000000711 ) ;
#4425=ORIENTED_EDGE ( 'NONE', *, *, #12842, .F. ) ;
#4437=DIRECTION ( 'NONE',  ( 0.000000000000000000, 0.000000000000000000, -1.000000000000000000 ) ) ;
#4460=EDGE_LOOP ( 'NONE', ( #4182, #1228, #1093, #1757, #5956, #11970, #2888, #10877, #11819 ) ) ;
#4470=CARTESIAN_POINT ( 'NONE',  ( 44.82050807568875683, 0.000000000000000000, 37.63139720814412925 ) ) ;
#4473=DIRECTION ( 'NONE',  ( -0.8660254037844387076, 0.000000000000000000, 0.4999999999999997224 ) ) ;
#4501=ORIENTED_EDGE ( 'NONE', *, *, #3581, .T. ) ;
#4509=DIRECTION ( 'NONE',  ( 0.000000000000000000, 0.000000000000000000, -1.000000000000000000 ) ) ;
#4516=ORIENTED_EDGE ( 'NONE', *, *, #4313, .F. ) ;
#4540=VERTEX_POINT ( 'NONE', #12403 ) ;
#4547=VECTOR ( 'NONE', #6917, 1000.000000000000000 ) ;
#4556=CARTESIAN_POINT ( 'NONE',  ( 14.41154273188008439, 88.59290746114278647, 60.96152422706632024 ) ) ;
#4558=LINE ( 'NONE', #8370, #4547 ) ;
#4568=PLANE ( 'NONE',  #4320 ) ;
#4570=LINE ( 'NONE', #9505, #7053 ) ;
#4576=ORIENTED_EDGE ( 'NONE', *, *, #475, .F. ) ;
#4578=ORIENTED_EDGE ( 'NONE', *, *, #7311, .T. ) ;
#4583=DIRECTION ( 'NONE',  ( -0.8660254037844388186, 0.000000000000000000, 0.4999999999999997780 ) ) ;
#4591=CARTESIAN_POINT ( 'NONE',  ( -60.00000000000000000, -37.00000000000000711, -20.00000000000000711 ) ) ;
#4592=CARTESIAN_POINT ( 'NONE',  ( 39.53738644056385709, 0.000000000000000000, 28.48076211354143794 ) ) ;
#4616=CYLINDRICAL_SURFACE ( 'NONE', #3572, 2.000000000000001332 ) ;
#4621=AXIS2_PLACEMENT_3D ( 'NONE', #14233, #2988, #7941 ) ;
#4627=VERTEX_POINT ( 'NONE', #702 ) ;
#4630=ORIENTED_EDGE ( 'NONE', *, *, #8121, .T. ) ;
#4638=DIRECTION ( 'NONE',  ( 1.000000000000000000, 0.000000000000000000, 0.000000000000000000 ) ) ;
#4639=EDGE_CURVE ( 'NONE', #4331, #13609, #15498, .T. ) ;
#4642=VERTEX_POINT ( 'NONE', #14022 ) ;
#4644=VECTOR ( 'NONE', #6675, 1000.000000000000000 ) ;
#4646=DIRECTION ( 'NONE',  ( -0.8660254037844388186, 0.000000000000000000, 0.4999999999999997780 ) ) ;
#4657=CARTESIAN_POINT ( 'NONE',  ( 42.02221399786069611, -3.000000000000000000, 2.650000000000096723 ) ) ;
#4659=ORIENTED_EDGE ( 'NONE', *, *, #275, .F. ) ;
#4666=CARTESIAN_POINT ( 'NONE',  ( 31.75426480542500229, -5.000000000000000000, -14.99999999999233324 ) ) ;
#4671=LINE ( 'NONE', #3379, #2942 ) ;
#4674=ORIENTED_EDGE ( 'NONE', *, *, #6006, .F. ) ;
#4677=ORIENTED_EDGE ( 'NONE', *, *, #3307, .F. ) ;
#4679=EDGE_CURVE ( 'NONE', #5955, #1559, #13318, .T. ) ;
#4683=DIRECTION ( 'NONE',  ( 0.8660254037844383745, 0.000000000000000000, 0.5000000000000005551 ) ) ;
#4693=VECTOR ( 'NONE', #15698, 1000.000000000000000 ) ;
#4710=CARTESIAN_POINT ( 'NONE',  ( 44.82050807568875683, -5.000000000000000000, 37.63139720814412925 ) ) ;
#4725=EDGE_CURVE ( 'NONE', #8017, #11683, #782, .T. ) ;
#4732=ORIENTED_EDGE ( 'NONE', *, *, #7757, .F. ) ;
#4737=EDGE_LOOP ( 'NONE', ( #9222, #6497, #6815, #15565, #4308, #8587, #1852, #15680 ) ) ;
#4745=CARTESIAN_POINT ( 'NONE',  ( 4.896370289181508184, -4.730053418719346148, 48.48076211353311749 ) ) ;
#4748=CARTESIAN_POINT ( 'NONE',  ( -2.886751345948139758, -37.00000000000000711, 35.00000000000000000 ) ) ;
#4774=CARTESIAN_POINT ( 'NONE',  ( 12.67949192431126093, -35.00000000000000000, -61.96152422706632024 ) ) ;
#4781=VECTOR ( 'NONE', #3264, 1000.000000000000000 ) ;
#4782=EDGE_LOOP ( 'NONE', ( #15079, #5900, #6570, #4674 ) ) ;
#4794=CARTESIAN_POINT ( 'NONE',  ( 4.896370289192182312, -5.000000000000000000, -48.48076211352908871 ) ) ;
#4808=CARTESIAN_POINT ( 'NONE',  ( 47.32050807568875683, -4.999999999999997335, 41.96152422706633445 ) ) ;
#4816=DIRECTION ( 'NONE',  ( -0.8660254037844387076, 0.000000000000000000, 0.4999999999999998335 ) ) ;
#4826=AXIS2_PLACEMENT_3D ( 'NONE', #954, #10884, #5882 ) ;
#4829=CARTESIAN_POINT ( 'NONE',  ( 42.02221399786069611, 0.000000000000000000, -2.649999999999888445 ) ) ;
#4838=ORIENTED_EDGE ( 'NONE', *, *, #9269, .F. ) ;
#4844=ADVANCED_FACE ( 'NONE', ( #6101 ), #4568, .F. ) ;
#4850=CARTESIAN_POINT ( 'NONE',  ( -28.86751345948126257, -4.999999999999997335, -50.00000000000000711 ) ) ;
#4856=CARTESIAN_POINT ( 'NONE',  ( 44.82050807568875683, 0.000000000000000000, 37.63139720814412925 ) ) ;
#4871=AXIS2_PLACEMENT_3D ( 'NONE', #4316, #3107, #764 ) ;
#4886=VECTOR ( 'NONE', #6814, 1000.000000000000114 ) ;
#4892=CARTESIAN_POINT ( 'NONE',  ( 45.58845726811988897, -35.00000000000000000, 42.96152422706634155 ) ) ;
#4898=CARTESIAN_POINT ( 'NONE',  ( 45.58845726811991739, -35.00000000000000000, -42.96152422706631313 ) ) ;
#4900=ORIENTED_EDGE ( 'NONE', *, *, #13733, .T. ) ;
#4929=CARTESIAN_POINT ( 'NONE',  ( 43.08845726811987475, 0.000000000000000000, 38.63139720814412925 ) ) ;
#4934=CARTESIAN_POINT ( 'NONE',  ( 12.67949192431120586, -37.00000000000000711, 61.96152422706632024 ) ) ;
#4943=CARTESIAN_POINT ( 'NONE',  ( 40.79973832332031236, -3.012258285427884541, 27.17844299114864626 ) ) ;
#4959=CARTESIAN_POINT ( 'NONE',  ( -1.154700538379222596, 88.59290746114278647, -34.00000000000000000 ) ) ;
#4962=ADVANCED_FACE ( 'NONE', ( #14913 ), #2610, .F. ) ;
#4991=CYLINDRICAL_SURFACE ( 'NONE', #2719, 2.649999999999992806 ) ;
#4996=CARTESIAN_POINT ( 'NONE',  ( -28.86751345948126612, -5.000000000000000000, -22.00000000000000711 ) ) ;
#5000=EDGE_CURVE ( 'NONE', #12993, #742, #5132, .T. ) ;
#5011=FILL_AREA_STYLE_COLOUR ( '', #7644 ) ;
#5012=ORIENTED_EDGE ( 'NONE', *, *, #10875, .T. ) ;
#5021=CIRCLE ( 'NONE', #7622, 32.00000000000000711 ) ;
#5035=DIRECTION ( 'NONE',  ( 0.000000000000000000, 0.000000000000000000, 1.000000000000000000 ) ) ;
#5037=ORIENTED_EDGE ( 'NONE', *, *, #8486, .F. ) ;
#5042=DIRECTION ( 'NONE',  ( -0.5000000000000005551, 0.000000000000000000, 0.8660254037844382635 ) ) ;
#5045=VECTOR ( 'NONE', #13460, 1000.000000000000000 ) ;
#5058=ORIENTED_EDGE ( 'NONE', *, *, #14714, .F. ) ;
#5067=DIRECTION ( 'NONE',  ( -0.5000000000000005551, 0.000000000000000000, 0.8660254037844382635 ) ) ;
#5073=AXIS2_PLACEMENT_3D ( 'NONE', #2870, #2705, #7663 ) ;
#5077=EDGE_LOOP ( 'NONE', ( #890, #9771, #11022, #8340 ) ) ;
#5078=EDGE_LOOP ( 'NONE', ( #5037, #9987, #4732, #5385, #4370, #12821, #9419, #3385 ) ) ;
#5086=VECTOR ( 'NONE', #13815, 1000.000000000000114 ) ;
#5091=DIRECTION ( 'NONE',  ( 0.000000000000000000, 1.000000000000000000, 0.000000000000000000 ) ) ;
#5092=CIRCLE ( 'NONE', #14131, 30.00000000000000711 ) ;
#5103=CARTESIAN_POINT ( 'NONE',  ( 10.17949192431125915, 0.000000000000000000, -57.63139720814413636 ) ) ;
#5115=DIRECTION ( 'NONE',  ( 0.8660254037844384856, -0.000000000000000000, 0.5000000000000004441 ) ) ;
#5120=FILL_AREA_STYLE_COLOUR ( '', #6856 ) ;
#5124=CIRCLE ( 'NONE', #1502, 2.000000000000001776 ) ;
#5132=LINE ( 'NONE', #12384, #14645 ) ;
#5148=ORIENTED_EDGE ( 'NONE', *, *, #1094, .T. ) ;
#5149=AXIS2_PLACEMENT_3D ( 'NONE', #9603, #13305, #7201 ) ;
#5152=CARTESIAN_POINT ( 'NONE',  ( -28.86751345948126257, -35.00000000000000000, -50.00000000000000711 ) ) ;
#5157=AXIS2_PLACEMENT_3D ( 'NONE', #1390, #14812, #12378 ) ;
#5180=CARTESIAN_POINT ( 'NONE',  ( 4.896370289181586344, 0.000000000000000000, 48.48076211353308906 ) ) ;
#5183=ORIENTED_EDGE ( 'NONE', *, *, #2547, .F. ) ;
#5186=CARTESIAN_POINT ( 'NONE',  ( 12.67949192431120586, 0.000000000000000000, 61.96152422706632024 ) ) ;
#5187=ORIENTED_EDGE ( 'NONE', *, *, #6405, .T. ) ;
#5207=DIRECTION ( 'NONE',  ( 0.000000000000000000, -0.000000000000000000, 1.000000000000000000 ) ) ;
#5213=DIRECTION ( 'NONE',  ( 0.000000000000000000, 0.000000000000000000, 1.000000000000000000 ) ) ;
#5216=ORIENTED_EDGE ( 'NONE', *, *, #734, .F. ) ;
#5230=LINE ( 'NONE', #15089, #6926 ) ;
#5233=EDGE_LOOP ( 'NONE', ( #15663, #2764 ) ) ;
#5239=VERTEX_POINT ( 'NONE', #9404 ) ;
#5255=( LENGTH_UNIT ( ) NAMED_UNIT ( * ) SI_UNIT ( .MILLI., .METRE. ) );
#5259=CARTESIAN_POINT ( 'NONE',  ( -44.40593521050208636, -4.342938577512204468, 20.10634714468941908 ) ) ;
#5271=CARTESIAN_POINT ( 'NONE',  ( 4.882921219558935988, -4.732646668675131174, -48.48447359618705121 ) ) ;
#5272=( LENGTH_UNIT ( ) NAMED_UNIT ( * ) SI_UNIT ( .MILLI., .METRE. ) );
#5275=DIRECTION ( 'NONE',  ( -8.673617379884037444E-16, 0.000000000000000000, -1.000000000000000000 ) ) ;
#5289=PLANE ( 'NONE',  #6859 ) ;
#5319=ORIENTED_EDGE ( 'NONE', *, *, #8718, .F. ) ;
#5322=AXIS2_PLACEMENT_3D ( 'NONE', #12904, #5719, #5487 ) ;
#5326=ORIENTED_EDGE ( 'NONE', *, *, #6221, .F. ) ;
#5340=EDGE_CURVE ( 'NONE', #715, #2379, #5092, .T. ) ;
#5347=CARTESIAN_POINT ( 'NONE',  ( -44.01413460128225807, -3.061199086701614114, 21.49255004891554677 ) ) ;
#5358=DIRECTION ( 'NONE',  ( 0.5000000000000002220, -1.734723475976806503E-15, 0.8660254037844383745 ) ) ;
#5370=CIRCLE ( 'NONE', #1754, 32.00000000000000711 ) ;
#5379=ADVANCED_FACE ( 'NONE', ( #14117 ), #10484, .F. ) ;
#5380=AXIS2_PLACEMENT_3D ( 'NONE', #6254, #6496, #8681 ) ;
#5381=DIRECTION ( 'NONE',  ( 0.000000000000000000, 0.000000000000000000, 1.000000000000000000 ) ) ;
#5385=ORIENTED_EDGE ( 'NONE', *, *, #11619, .F. ) ;
#5388=CIRCLE ( 'NONE', #6419, 32.00000000000000711 ) ;
#5420=CARTESIAN_POINT ( 'NONE',  ( -44.21674811821717554, -3.395032785697067901, -20.79966053514407420 ) ) ;
#5426=VERTEX_POINT ( 'NONE', #3199 ) ;
#5427=ORIENTED_EDGE ( 'NONE', *, *, #3362, .F. ) ;
#5453=LINE ( 'NONE', #4400, #3871 ) ;
#5456=EDGE_LOOP ( 'NONE', ( #15248, #2749, #9377, #11898 ) ) ;
#5459=DIRECTION ( 'NONE',  ( -0.000000000000000000, 1.000000000000000000, -0.000000000000000000 ) ) ;
#5487=DIRECTION ( 'NONE',  ( 0.000000000000000000, 0.000000000000000000, -1.000000000000000000 ) ) ;
#5505=AXIS2_PLACEMENT_3D ( 'NONE', #2063, #8228, #13126 ) ;
#5530=CARTESIAN_POINT ( 'NONE',  ( -60.00000000000000000, 0.000000000000000000, -18.00000000000001066 ) ) ;
#5539=ORIENTED_EDGE ( 'NONE', *, *, #600, .T. ) ;
#5547=DIRECTION ( 'NONE',  ( 0.4999999999999997224, 0.000000000000000000, 0.8660254037844388186 ) ) ;
#5552=CARTESIAN_POINT ( 'NONE',  ( -28.86751345948129455, -3.000000000000000000, 49.99999999999999289 ) ) ;
#5556=ORIENTED_EDGE ( 'NONE', *, *, #8574, .T. ) ;
#5567=ORIENTED_EDGE ( 'NONE', *, *, #1571, .F. ) ;
#5569=CARTESIAN_POINT ( 'NONE',  ( 45.58845726811988897, 88.59290746114278647, 42.96152422706634155 ) ) ;
#5578=AXIS2_PLACEMENT_3D ( 'NONE', #2748, #14064, #9150 ) ;
#5588=CYLINDRICAL_SURFACE ( 'NONE', #1916, 39.99999999999999289 ) ;
#5590=CARTESIAN_POINT ( 'NONE',  ( 40.89003422689814471, -3.000000000000000000, -27.08062585941929967 ) ) ;
#5607=CARTESIAN_POINT ( 'NONE',  ( 39.54732521363962405, -4.732646668676187218, 28.47097061891900438 ) ) ;
#5612=DIRECTION ( 'NONE',  ( -0.8660254037844385966, 0.000000000000000000, -0.5000000000000000000 ) ) ;
#5627=EDGE_CURVE ( 'NONE', #2457, #8017, #8514, .T. ) ;
#5630=ADVANCED_FACE ( 'NONE', ( #15937 ), #13244, .T. ) ;
#5640=LINE ( 'NONE', #4657, #11760 ) ;
#5651=CARTESIAN_POINT ( 'NONE',  ( 3.007492831193109062, -2.999999999999999556, 48.95212133182432268 ) ) ;
#5652=AXIS2_PLACEMENT_3D ( 'NONE', #4850, #11949, #12262 ) ;
#5666=DIRECTION ( 'NONE',  ( -0.5000000000000005551, 0.000000000000000000, 0.8660254037844383745 ) ) ;
#5667=VERTEX_POINT ( 'NONE', #11955 ) ;
#5668=CARTESIAN_POINT ( 'NONE',  ( -60.00000000000000000, -5.000000000000004441, 17.99999999999999289 ) ) ;
#5676=PRODUCT_CONTEXT ( 'NONE', #7320, 'mechanical' ) ;
#5681=DIRECTION ( 'NONE',  ( -1.000000000000000000, 0.000000000000000000, -3.343241100358131282E-16 ) ) ;
#5682=EDGE_LOOP ( 'NONE', ( #5856, #8565, #5697, #359 ) ) ;
#5689=LINE ( 'NONE', #4151, #1238 ) ;
#5693=DIRECTION ( 'NONE',  ( 1.000000000000000000, 1.734723475976808080E-15, 0.000000000000000000 ) ) ;
#5697=ORIENTED_EDGE ( 'NONE', *, *, #8121, .F. ) ;
#5719=DIRECTION ( 'NONE',  ( 0.000000000000000000, -1.000000000000000000, 0.000000000000000000 ) ) ;
#5732=ORIENTED_EDGE ( 'NONE', *, *, #9551, .F. ) ;
#5743=CARTESIAN_POINT ( 'NONE',  ( 40.27815445939820904, -3.253774389711718396, -27.73097106845637683 ) ) ;
#5755=AXIS2_PLACEMENT_3D ( 'NONE', #7364, #10030, #9697 ) ;
#5761=CARTESIAN_POINT ( 'NONE',  ( -5.725490332117410652, -3.000000000000000000, 49.91684015347181003 ) ) ;
#5773=LINE ( 'NONE', #13659, #14626 ) ;
#5784=VECTOR ( 'NONE', #1845, 1000.000000000000000 ) ;
#5786=ORIENTED_EDGE ( 'NONE', *, *, #8574, .F. ) ;
#5808=AXIS2_PLACEMENT_3D ( 'NONE', #9615, #10683, #9470 ) ;
#5818=CARTESIAN_POINT ( 'NONE',  ( -1.154700538379217711, -35.00000000000000000, -34.00000000000000000 ) ) ;
#5822=AXIS2_PLACEMENT_3D ( 'NONE', #662, #5666, #12997 ) ;
#5829=ORIENTED_EDGE ( 'NONE', *, *, #12191, .T. ) ;
#5836=ORIENTED_EDGE ( 'NONE', *, *, #10295, .T. ) ;
#5848=DIRECTION ( 'NONE',  ( 0.000000000000000000, 1.000000000000000000, 0.000000000000000000 ) ) ;
#5854=CIRCLE ( 'NONE', #14114, 2.000000000000000000 ) ;
#5856=ORIENTED_EDGE ( 'NONE', *, *, #12929, .F. ) ;
#5882=DIRECTION ( 'NONE',  ( 0.000000000000000000, 0.000000000000000000, -1.000000000000000000 ) ) ;
#5896=LINE ( 'NONE', #2476, #7983 ) ;
#5900=ORIENTED_EDGE ( 'NONE', *, *, #9965, .F. ) ;
#5938=ORIENTED_EDGE ( 'NONE', *, *, #13620, .F. ) ;
#5947=DIRECTION ( 'NONE',  ( -0.000000000000000000, 1.000000000000000000, -0.000000000000000000 ) ) ;
#5954=FACE_OUTER_BOUND ( 'NONE', #8604, .T. ) ;
#5955=VERTEX_POINT ( 'NONE', #4075 ) ;
#5956=ORIENTED_EDGE ( 'NONE', *, *, #10861, .T. ) ;
#5959=LINE ( 'NONE', #15822, #11281 ) ;
#5969=LINE ( 'NONE', #3691, #7717 ) ;
#5974=ORIENTED_EDGE ( 'NONE', *, *, #3382, .F. ) ;
#5983=CARTESIAN_POINT ( 'NONE',  ( -5.725490332117410652, -3.000000000000000000, 9.916840153471811803 ) ) ;
#5993=EDGE_CURVE ( 'NONE', #8265, #15092, #13093, .T. ) ;
#5996=VERTEX_POINT ( 'NONE', #6353 ) ;
#5999=CARTESIAN_POINT ( 'NONE',  ( -5.725490332106780933, -3.000000000000000000, -9.916840153467775920 ) ) ;
#6000=CIRCLE ( 'NONE', #13731, 30.00000000000000711 ) ;
#6006=EDGE_CURVE ( 'NONE', #15603, #12752, #12469, .T. ) ;
#6013=VECTOR ( 'NONE', #13724, 1000.000000000000000 ) ;
#6016=AXIS2_PLACEMENT_3D ( 'NONE', #7927, #15106, #10184 ) ;
#6025=EDGE_CURVE ( 'NONE', #13521, #2121, #7656, .T. ) ;
#6056=DIRECTION ( 'NONE',  ( 0.000000000000000000, 0.000000000000000000, 1.000000000000000000 ) ) ;
#6057=VECTOR ( 'NONE', #664, 1000.000000000000227 ) ;
#6064=LINE ( 'NONE', #8580, #12423 ) ;
#6074=B_SPLINE_CURVE_WITH_KNOTS ( 'NONE', 3,
 ( #11773, #5651, #13066, #10594, #15518, #6953, #11855, #803, #14373, #7504, #2232, #15907, #6126, #15827, #4745, #65 ),
 .UNSPECIFIED., .F., .F.,
 ( 4, 2, 2, 2, 2, 2, 2, 4 ),
 ( 1.371419323662773723E-18, 0.0003988081628697417893, 0.0007976163257394822776, 0.001196424488609222712, 0.001595232651478961953, 0.001994040814348701195, 0.002392848977218440219, 0.003190465302957923906 ),
 .UNSPECIFIED. ) ;
#6079=EDGE_CURVE ( 'NONE', #10036, #7945, #690, .T. ) ;
#6080=CARTESIAN_POINT ( 'NONE',  ( -2.886751345948099789, 0.000000000000000000, -35.00000000000000000 ) ) ;
#6096=ADVANCED_FACE ( 'NONE', ( #14259 ), #6680, .F. ) ;
#6098=VECTOR ( 'NONE', #2967, 1000.000000000000000 ) ;
#6101=FACE_OUTER_BOUND ( 'NONE', #3099, .T. ) ;
#6125=FACE_OUTER_BOUND ( 'NONE', #478, .T. ) ;
#6126=CARTESIAN_POINT ( 'NONE',  ( 4.686367213310268731, -4.097106062772740920, 48.53802711916877399 ) ) ;
#6160=ORIENTED_EDGE ( 'NONE', *, *, #205, .F. ) ;
#6164=CIRCLE ( 'NONE', #5652, 30.00000000000000711 ) ;
#6169=DIRECTION ( 'NONE',  ( 0.000000000000000000, 0.000000000000000000, 1.000000000000000000 ) ) ;
#6176=CARTESIAN_POINT ( 'NONE',  ( 30.02221399786052913, 0.000000000000000000, 16.00000000000001066 ) ) ;
#6194=CARTESIAN_POINT ( 'NONE',  ( -1.154700538379255903, 0.000000000000000000, 34.00000000000000711 ) ) ;
#6200=EDGE_CURVE ( 'NONE', #1559, #12752, #5124, .T. ) ;
#6202=EDGE_LOOP ( 'NONE', ( #15329, #12599, #9206, #13995, #24, #1556, #13140, #1631 ) ) ;
#6207=DIRECTION ( 'NONE',  ( 0.000000000000000000, -1.000000000000000000, 0.000000000000000000 ) ) ;
#6208=CARTESIAN_POINT ( 'NONE',  ( 57.73502691896258199, -35.00000000000000000, 2.081668171172168513E-14 ) ) ;
#6210=CARTESIAN_POINT ( 'NONE',  ( -55.00000000000000000, -5.000000000000000000, 19.99999999999999289 ) ) ;
#6220=VERTEX_POINT ( 'NONE', #2430 ) ;
#6221=EDGE_CURVE ( 'NONE', #11703, #15563, #3656, .T. ) ;
#6227=DIRECTION ( 'NONE',  ( 0.000000000000000000, 0.000000000000000000, -1.000000000000000000 ) ) ;
#6228=FACE_OUTER_BOUND ( 'NONE', #11956, .T. ) ;
#6243=DIRECTION ( 'NONE',  ( 0.000000000000000000, 0.000000000000000000, 1.000000000000000000 ) ) ;
#6246=CARTESIAN_POINT ( 'NONE',  ( 40.27451087355422743, -3.242827243955479943, 27.73563889972393426 ) ) ;
#6254=CARTESIAN_POINT ( 'NONE',  ( -5.725490332117410652, 0.000000000000000000, 9.916840153471811803 ) ) ;
#6258=DIRECTION ( 'NONE',  ( -0.8660254037844387076, -0.000000000000000000, 0.4999999999999997224 ) ) ;
#6283=AXIS2_PLACEMENT_3D ( 'NONE', #2008, #7031, #4437 ) ;
#6284=CARTESIAN_POINT ( 'NONE',  ( -44.43375672974055846, 0.000000000000000000, 19.99999999999999645 ) ) ;
#6285=VECTOR ( 'NONE', #15408, 1000.000000000000000 ) ;
#6296=CIRCLE ( 'NONE', #12460, 27.99999999999998934 ) ;
#6297=DIRECTION ( 'NONE',  ( -0.8660254037844387076, -0.000000000000000000, 0.4999999999999997224 ) ) ;
#6311=CARTESIAN_POINT ( 'NONE',  ( -2.886751345948099789, -4.999999999999997335, -35.00000000000000000 ) ) ;
#6317=ORIENTED_EDGE ( 'NONE', *, *, #13380, .T. ) ;
#6319=VERTEX_POINT ( 'NONE', #8599 ) ;
#6341=EDGE_CURVE ( 'NONE', #7945, #14772, #10783, .T. ) ;
#6344=DIRECTION ( 'NONE',  ( -0.000000000000000000, 1.000000000000000000, -0.000000000000000000 ) ) ;
#6353=CARTESIAN_POINT ( 'NONE',  ( 33.48631561299829684, -3.000000000000000000, 14.00000000000000888 ) ) ;
#6365=CARTESIAN_POINT ( 'NONE',  ( -43.85680617778868395, -3.000000000000000000, -22.00000000000000355 ) ) ;
#6383=CYLINDRICAL_SURFACE ( 'NONE', #2994, 31.99999999999999289 ) ;
#6389=CYLINDRICAL_SURFACE ( 'NONE', #3946, 2.649999999999992806 ) ;
#6404=PLANE ( 'NONE',  #5578 ) ;
#6405=EDGE_CURVE ( 'NONE', #8017, #2243, #15218, .T. ) ;
#6411=CARTESIAN_POINT ( 'NONE',  ( -55.00000000000000000, 0.000000000000000000, -18.00000000000001066 ) ) ;
#6416=FACE_OUTER_BOUND ( 'NONE', #2147, .T. ) ;
#6417=ORIENTED_EDGE ( 'NONE', *, *, #4639, .F. ) ;
#6419=AXIS2_PLACEMENT_3D ( 'NONE', #13341, #5848, #13256 ) ;
#6429=AXIS2_PLACEMENT_3D ( 'NONE', #1358, #8974, #10020 ) ;
#6434=VECTOR ( 'NONE', #12164, 1000.000000000000000 ) ;
#6440=CARTESIAN_POINT ( 'NONE',  ( -5.725490332117410652, -3.000000000000000000, 9.916840153471811803 ) ) ;
#6441=DIRECTION ( 'NONE',  ( 0.000000000000000000, -0.000000000000000000, -1.000000000000000000 ) ) ;
#6445=EDGE_CURVE ( 'NONE', #742, #14284, #11807, .T. ) ;
#6463=ORIENTED_EDGE ( 'NONE', *, *, #3631, .T. ) ;
#6479=ORIENTED_EDGE ( 'NONE', *, *, #3613, .T. ) ;
#6486=B_SPLINE_CURVE_WITH_KNOTS ( 'NONE', 3,
 ( #3159, #5590, #3394, #978, #900, #15610, #5743, #10527, #12924, #15461, #14397, #2176, #15775, #4382, #6805, #9316 ),
 .UNSPECIFIED., .F., .F.,
 ( 4, 2, 2, 2, 2, 2, 2, 4 ),
 ( 0.000000000000000000, 0.0003988081628697240084, 0.0007976163257394480169, 0.001196424488609171971, 0.001595232651478896034, 0.001994040814348619229, 0.002392848977218342207, 0.003190465302957785562 ),
 .UNSPECIFIED. ) ;
#6496=DIRECTION ( 'NONE',  ( 0.000000000000000000, -1.000000000000000000, 0.000000000000000000 ) ) ;
#6497=ORIENTED_EDGE ( 'NONE', *, *, #15255, .T. ) ;
#6517=ORIENTED_EDGE ( 'NONE', *, *, #7135, .F. ) ;
#6536=VERTEX_POINT ( 'NONE', #12112 ) ;
#6539=EDGE_LOOP ( 'NONE', ( #999, #14173, #254, #5326, #11140, #1636, #5148 ) ) ;
#6558=CARTESIAN_POINT ( 'NONE',  ( -44.36165667912468535, -3.982459619754737723, 20.27312360634764232 ) ) ;
#6561=DIRECTION ( 'NONE',  ( 0.000000000000000000, 0.000000000000000000, 1.000000000000000000 ) ) ;
#6566=AXIS2_PLACEMENT_3D ( 'NONE', #13220, #2159, #3450 ) ;
#6570=ORIENTED_EDGE ( 'NONE', *, *, #6200, .T. ) ;
#6571=CARTESIAN_POINT ( 'NONE',  ( 31.75426480542942898, -37.00000000000000711, -14.99999999999999645 ) ) ;
#6588=VECTOR ( 'NONE', #8378, 1000.000000000000000 ) ;
#6601=PLANE ( 'NONE',  #3214 ) ;
#6612=AXIS2_PLACEMENT_3D ( 'NONE', #6853, #3511, #11762 ) ;
#6626=DIRECTION ( 'NONE',  ( 0.000000000000000000, -1.000000000000000000, 0.000000000000000000 ) ) ;
#6637=CARTESIAN_POINT ( 'NONE',  ( -60.00000000000000000, 88.59290746114278647, 17.99999999999999289 ) ) ;
#6642=ORIENTED_EDGE ( 'NONE', *, *, #205, .T. ) ;
#6660=VECTOR ( 'NONE', #6789, 1000.000000000000000 ) ;
#6667=VECTOR ( 'NONE', #8942, 1000.000000000000227 ) ;
#6675=DIRECTION ( 'NONE',  ( -0.000000000000000000, 1.000000000000000000, -0.000000000000000000 ) ) ;
#6680=PLANE ( 'NONE',  #6921 ) ;
#6693=FACE_OUTER_BOUND ( 'NONE', #1930, .T. ) ;
#6695=DIRECTION ( 'NONE',  ( 0.000000000000000000, 0.000000000000000000, 1.000000000000000000 ) ) ;
#6711=VERTEX_POINT ( 'NONE', #44 ) ;
#6713=CIRCLE ( 'NONE', #3820, 5.000000000000001776 ) ;
#6727=ORIENTED_EDGE ( 'NONE', *, *, #1950, .F. ) ;
#6729=CARTESIAN_POINT ( 'NONE',  ( 39.53738644056090124, -3.000000000000000000, 28.48076211354432985 ) ) ;
#6746=ORIENTED_EDGE ( 'NONE', *, *, #1574, .T. ) ;
#6758=DIRECTION ( 'NONE',  ( 0.000000000000000000, -1.000000000000000000, 0.000000000000000000 ) ) ;
#6768=FACE_OUTER_BOUND ( 'NONE', #5456, .T. ) ;
#6783=AXIS2_PLACEMENT_3D ( 'NONE', #6210, #2387, #9907 ) ;
#6789=DIRECTION ( 'NONE',  ( 0.000000000000000000, -1.000000000000000000, 0.000000000000000000 ) ) ;
#6795=ORIENTED_EDGE ( 'NONE', *, *, #8718, .T. ) ;
#6798=CIRCLE ( 'NONE', #6016, 2.649999999999985700 ) ;
#6805=CARTESIAN_POINT ( 'NONE',  ( 39.53738644055563611, -4.730053418719265323, -28.48076211352709564 ) ) ;
#6807=LINE ( 'NONE', #9157, #7545 ) ;
#6814=DIRECTION ( 'NONE',  ( 0.4999999999999998335, -0.000000000000000000, 0.8660254037844387076 ) ) ;
#6815=ORIENTED_EDGE ( 'NONE', *, *, #9985, .T. ) ;
#6853=CARTESIAN_POINT ( 'NONE',  ( -21.01110699893060030, -3.000000000000001332, 36.39230484541324273 ) ) ;
#6856=COLOUR_RGB ( '', 0.09019608, 0.27058824, 0.51372549) ;
#6859=AXIS2_PLACEMENT_3D ( 'NONE', #3022, #13852, #10385 ) ;
#6864=DIRECTION ( 'NONE',  ( -0.000000000000000000, 1.000000000000000000, -0.000000000000000000 ) ) ;
#6867=DIRECTION ( 'NONE',  ( -0.000000000000000000, 1.000000000000000000, -0.000000000000000000 ) ) ;
#6871=FACE_OUTER_BOUND ( 'NONE', #12582, .T. ) ;
#6878=EDGE_CURVE ( 'NONE', #1232, #10374, #1720, .T. ) ;
#6880=ORIENTED_EDGE ( 'NONE', *, *, #10177, .T. ) ;
#6892=VECTOR ( 'NONE', #9666, 1000.000000000000000 ) ;
#6897=EDGE_LOOP ( 'NONE', ( #3624, #3189, #4425, #11341, #14973, #13010, #15184, #6160, #11171, #6970, #285, #14481 ) ) ;
#6901=LINE ( 'NONE', #14482, #11844 ) ;
#6902=ORIENTED_EDGE ( 'NONE', *, *, #5627, .F. ) ;
#6915=DIRECTION ( 'NONE',  ( 1.000000000000000000, -0.000000000000000000, 0.000000000000000000 ) ) ;
#6917=DIRECTION ( 'NONE',  ( 0.000000000000000000, 0.000000000000000000, -1.000000000000000000 ) ) ;
#6921=AXIS2_PLACEMENT_3D ( 'NONE', #3187, #1809, #14187 ) ;
#6926=VECTOR ( 'NONE', #14028, 1000.000000000000000 ) ;
#6932=CARTESIAN_POINT ( 'NONE',  ( 12.67949192431126093, -37.00000000000000711, -61.96152422706632024 ) ) ;
#6940=VERTEX_POINT ( 'NONE', #4470 ) ;
#6949=CIRCLE ( 'NONE', #12809, 2.649999999999992806 ) ;
#6953=CARTESIAN_POINT ( 'NONE',  ( 3.761221015330621587, -3.194220869028280507, 48.77578944492238833 ) ) ;
#6970=ORIENTED_EDGE ( 'NONE', *, *, #8773, .F. ) ;
#6978=DIRECTION ( 'NONE',  ( 0.000000000000000000, -1.000000000000000000, 0.000000000000000000 ) ) ;
#6981=SHAPE_REPRESENTATION ( 'Precision Linear Jaw Guides', ( #3223 ), #14881 ) ;
#6994=LINE ( 'NONE', #5530, #4781 ) ;
#7011=DIRECTION ( 'NONE',  ( 0.000000000000000000, -1.000000000000000000, 0.000000000000000000 ) ) ;
#7031=DIRECTION ( 'NONE',  ( -0.000000000000000000, -1.000000000000000000, -0.000000000000000000 ) ) ;
#7038=VERTEX_POINT ( 'NONE', #3178 ) ;
#7042=ORIENTED_EDGE ( 'NONE', *, *, #63, .F. ) ;
#7053=VECTOR ( 'NONE', #3197, 1000.000000000000000 ) ;
#7055=VERTEX_POINT ( 'NONE', #10694 ) ;
#7060=CIRCLE ( 'NONE', #5755, 30.00000000000000711 ) ;
#7074=EDGE_CURVE ( 'NONE', #3918, #12974, #11822, .T. ) ;
#7080=CYLINDRICAL_SURFACE ( 'NONE', #13473, 5.000000000000000000 ) ;
#7096=EDGE_CURVE ( 'NONE', #10415, #12974, #12064, .T. ) ;
#7103=AXIS2_PLACEMENT_3D ( 'NONE', #13773, #2871, #7580 ) ;
#7108=DIRECTION ( 'NONE',  ( -0.000000000000000000, 1.000000000000000000, -0.000000000000000000 ) ) ;
#7111=ORIENTED_EDGE ( 'NONE', *, *, #11437, .F. ) ;
#7115=ORIENTED_EDGE ( 'NONE', *, *, #11371, .F. ) ;
#7127=VECTOR ( 'NONE', #15456, 1000.000000000000114 ) ;
#7129=AXIS2_PLACEMENT_3D ( 'NONE', #743, #12923, #12999 ) ;
#7135=EDGE_CURVE ( 'NONE', #6319, #5667, #6949, .T. ) ;
#7144=LINE ( 'NONE', #6080, #1776 ) ;
#7153=EDGE_CURVE ( 'NONE', #11683, #12492, #7144, .T. ) ;
#7187=ADVANCED_FACE ( 'NONE', ( #12368, #2276 ), #1064, .F. ) ;
#7188=CARTESIAN_POINT ( 'NONE',  ( -4.618802153517020948, -3.000000000000000000, 36.00000000000000711 ) ) ;
#7201=DIRECTION ( 'NONE',  ( 0.000000000000000000, 0.000000000000000000, 1.000000000000000000 ) ) ;
#7204=CYLINDRICAL_SURFACE ( 'NONE', #8172, 1.999999999999998668 ) ;
#7220=AXIS2_PLACEMENT_3D ( 'NONE', #9266, #11137, #14192 ) ;
#7223=VERTEX_POINT ( 'NONE', #191 ) ;
#7228=CARTESIAN_POINT ( 'NONE',  ( 39.69153896976634144, -4.098233149437865208, 28.32796736983516794 ) ) ;
#7229=AXIS2_PLACEMENT_3D ( 'NONE', #11255, #11100, #7473 ) ;
#7234=ORIENTED_EDGE ( 'NONE', *, *, #5993, .T. ) ;
#7238=VERTEX_POINT ( 'NONE', #516 ) ;
#7247=DIRECTION ( 'NONE',  ( 0.4999999999999997224, 1.734723475976807094E-15, 0.8660254037844387076 ) ) ;
#7255=EDGE_LOOP ( 'NONE', ( #15509, #2416 ) ) ;
#7276=DIRECTION ( 'NONE',  ( -0.8660254037844381525, 0.000000000000000000, -0.5000000000000007772 ) ) ;
#7277=ORIENTED_EDGE ( 'NONE', *, *, #4313, .T. ) ;
#7278=CARTESIAN_POINT ( 'NONE',  ( 4.896370289181515290, -5.000000000000000000, 48.48076211353313170 ) ) ;
#7289=VERTEX_POINT ( 'NONE', #6411 ) ;
#7296=CARTESIAN_POINT ( 'NONE',  ( -1.154700538379218600, -35.00000000000000000, -34.00000000000000000 ) ) ;
#7311=EDGE_CURVE ( 'NONE', #5426, #5955, #15828, .T. ) ;
#7315=DIRECTION ( 'NONE',  ( -0.4999999999999998335, 0.000000000000000000, -0.8660254037844387076 ) ) ;
#7320=APPLICATION_CONTEXT ( 'automotive_design' ) ;
#7351=CARTESIAN_POINT ( 'NONE',  ( -5.725490332117410652, 0.000000000000000000, 9.916840153471811803 ) ) ;
#7363=VECTOR ( 'NONE', #9642, 1000.000000000000114 ) ;
#7364=CARTESIAN_POINT ( 'NONE',  ( -28.86751345948126257, -37.00000000000000711, -50.00000000000000711 ) ) ;
#7370=VECTOR ( 'NONE', #9454, 1000.000000000000000 ) ;
#7374=DIRECTION ( 'NONE',  ( -0.000000000000000000, 1.000000000000000000, 0.000000000000000000 ) ) ;
#7378=CIRCLE ( 'NONE', #13293, 2.000000000000000888 ) ;
#7389=EDGE_LOOP ( 'NONE', ( #11802, #3051 ) ) ;
#7401=CARTESIAN_POINT ( 'NONE',  ( 0.000000000000000000, 0.000000000000000000, 0.000000000000000000 ) ) ;
#7403=DIRECTION ( 'NONE',  ( -0.4999999999999997224, 8.673617379884035472E-16, -0.8660254037844387076 ) ) ;
#7416=CYLINDRICAL_SURFACE ( 'NONE', #3259, 5.000000000000000000 ) ;
#7424=CARTESIAN_POINT ( 'NONE',  ( 47.32050807568879947, -37.00000000000000711, -41.96152422706630603 ) ) ;
#7433=ORIENTED_EDGE ( 'NONE', *, *, #762, .T. ) ;
#7441=CARTESIAN_POINT ( 'NONE',  ( 44.82050807568879947, -5.000000000000000000, -37.63139720814411504 ) ) ;
#7445=LINE ( 'NONE', #9779, #1628 ) ;
#7461=CARTESIAN_POINT ( 'NONE',  ( 10.17949192431126093, 0.000000000000000000, -57.63139720814412925 ) ) ;
#7463=CARTESIAN_POINT ( 'NONE',  ( 40.62016163511525946, -3.061199086701585248, 27.37108366584844532 ) ) ;
#7470=ORIENTED_EDGE ( 'NONE', *, *, #14817, .T. ) ;
#7472=VERTEX_POINT ( 'NONE', #13621 ) ;
#7473=DIRECTION ( 'NONE',  ( 0.000000000000000000, 0.000000000000000000, 1.000000000000000000 ) ) ;
#7486=CARTESIAN_POINT ( 'NONE',  ( 47.32050807568880657, -5.000000000000000000, -41.96152422706630603 ) ) ;
#7504=CARTESIAN_POINT ( 'NONE',  ( 4.387887813791333080, -3.660959011663040386, 48.61734447228085543 ) ) ;
#7518=CARTESIAN_POINT ( 'NONE',  ( -28.86751345948129455, -37.00000000000000711, 20.00000000000000355 ) ) ;
#7532=DIRECTION ( 'NONE',  ( 0.000000000000000000, -1.000000000000000000, 0.000000000000000000 ) ) ;
#7534=ORIENTED_EDGE ( 'NONE', *, *, #3560, .F. ) ;
#7537=ORIENTED_EDGE ( 'NONE', *, *, #10397, .F. ) ;
#7539=CARTESIAN_POINT ( 'NONE',  ( 45.58845726811992449, -5.000000000000004441, -42.96152422706630603 ) ) ;
#7540=ADVANCED_FACE ( 'NONE', ( #10087 ), #388, .F. ) ;
#7545=VECTOR ( 'NONE', #9080, 1000.000000000000000 ) ;
#7553=CARTESIAN_POINT ( 'NONE',  ( -28.86751345948130165, 0.000000000000000000, 20.00000000000000355 ) ) ;
#7563=PRODUCT_DEFINITION_CONTEXT ( 'detailed design', #1125, 'design' ) ;
#7564=DIRECTION ( 'NONE',  ( -0.5000000000000005551, 0.000000000000000000, 0.8660254037844382635 ) ) ;
#7580=DIRECTION ( 'NONE',  ( 0.000000000000000000, 0.000000000000000000, -1.000000000000000000 ) ) ;
#7598=VECTOR ( 'NONE', #4473, 1000.000000000000114 ) ;
#7601=FACE_BOUND ( 'NONE', #2862, .T. ) ;
#7618=EDGE_LOOP ( 'NONE', ( #6795, #6642, #9515, #9455 ) ) ;
#7619=FACE_OUTER_BOUND ( 'NONE', #5682, .T. ) ;
#7622=AXIS2_PLACEMENT_3D ( 'NONE', #6208, #12161, #13211 ) ;
#7627=EDGE_CURVE ( 'NONE', #4627, #3387, #1823, .T. ) ;
#7634=CARTESIAN_POINT ( 'NONE',  ( 3.393972966170744510, -3.061199086701537286, -48.86363371475460582 ) ) ;
#7644=COLOUR_RGB ( '', 0.09019608, 0.27058824, 0.51372549) ;
#7647=VECTOR ( 'NONE', #14972, 1000.000000000000114 ) ;
#7649=FACE_BOUND ( 'NONE', #7255, .T. ) ;
#7653=DIRECTION ( 'NONE',  ( 0.000000000000000000, 0.000000000000000000, 1.000000000000000000 ) ) ;
#7656=LINE ( 'NONE', #3990, #6667 ) ;
#7661=ORIENTED_EDGE ( 'NONE', *, *, #7074, .F. ) ;
#7663=DIRECTION ( 'NONE',  ( 0.000000000000000000, 0.000000000000000000, 1.000000000000000000 ) ) ;
#7676=EDGE_LOOP ( 'NONE', ( #7234, #1332, #7871, #5216 ) ) ;
#7685=ADVANCED_FACE ( 'NONE', ( #6768 ), #12888, .T. ) ;
#7688=CIRCLE ( 'NONE', #9994, 31.99999999999999289 ) ;
#7693=CARTESIAN_POINT ( 'NONE',  ( -44.41942919302233150, -4.462727778340706664, -20.05540692447297246 ) ) ;
#7704=CARTESIAN_POINT ( 'NONE',  ( -44.37850886472753587, -4.098233149438287093, 20.20989737819990495 ) ) ;
#7705=ORIENTED_EDGE ( 'NONE', *, *, #13235, .T. ) ;
#7708=EDGE_CURVE ( 'NONE', #1994, #5239, #10332, .T. ) ;
#7717=VECTOR ( 'NONE', #10890, 1000.000000000000000 ) ;
#7721=SHAPE_REPRESENTATION_RELATIONSHIP ( 'NONE' , 'NONE' ,  #6981, #1740 ) ;
#7731=VECTOR ( 'NONE', #5947, 1000.000000000000000 ) ;
#7732=AXIS2_PLACEMENT_3D ( 'NONE', #13794, #10268, #8651 ) ;
#7735=PLANE ( 'NONE',  #492 ) ;
#7748=VECTOR ( 'NONE', #5681, 1000.000000000000000 ) ;
#7757=EDGE_CURVE ( 'NONE', #7238, #7869, #1014, .T. ) ;
#7786=CARTESIAN_POINT ( 'NONE',  ( -44.29799420005891619, -3.661800705855200899, 20.50793615625904209 ) ) ;
#7799=DIRECTION ( 'NONE',  ( 0.000000000000000000, 0.000000000000000000, -1.000000000000000000 ) ) ;
#7816=CARTESIAN_POINT ( 'NONE',  ( 57.73502691896258199, -4.999999999999997335, 2.081668171172168513E-14 ) ) ;
#7820=ORIENTED_EDGE ( 'NONE', *, *, #13990, .F. ) ;
#7823=FACE_OUTER_BOUND ( 'NONE', #4737, .T. ) ;
#7855=ORIENTED_EDGE ( 'NONE', *, *, #15532, .T. ) ;
#7857=VERTEX_POINT ( 'NONE', #11985 ) ;
#7862=EDGE_CURVE ( 'NONE', #4061, #10685, #1084, .T. ) ;
#7869=VERTEX_POINT ( 'NONE', #13127 ) ;
#7871=ORIENTED_EDGE ( 'NONE', *, *, #1378, .T. ) ;
#7876=CIRCLE ( 'NONE', #8916, 5.000000000000001776 ) ;
#7878=EDGE_CURVE ( 'NONE', #7055, #10036, #14940, .T. ) ;
#7886=DIRECTION ( 'NONE',  ( -0.000000000000000000, 1.000000000000000000, -0.000000000000000000 ) ) ;
#7887=FACE_OUTER_BOUND ( 'NONE', #6202, .T. ) ;
#7902=AXIS2_PLACEMENT_3D ( 'NONE', #7441, #4683, #8650 ) ;
#7905=DIRECTION ( 'NONE',  ( -0.000000000000000000, 1.000000000000000000, -0.000000000000000000 ) ) ;
#7922=ADVANCED_FACE ( 'NONE', ( #7649, #3907 ), #7735, .T. ) ;
#7924=CIRCLE ( 'NONE', #14843, 39.99999999999999289 ) ;
#7925=LINE ( 'NONE', #3215, #12866 ) ;
#7927=CARTESIAN_POINT ( 'NONE',  ( -21.01110699893041911, -3.000000000000001332, -36.39230484541334221 ) ) ;
#7930=CIRCLE ( 'NONE', #1461, 31.99999999999999289 ) ;
#7939=VECTOR ( 'NONE', #5547, 1000.000000000000114 ) ;
#7940=ORIENTED_EDGE ( 'NONE', *, *, #6221, .T. ) ;
#7941=DIRECTION ( 'NONE',  ( 9.912705577010324563E-16, 0.000000000000000000, 1.000000000000000000 ) ) ;
#7945=VERTEX_POINT ( 'NONE', #8853 ) ;
#7953=ORIENTED_EDGE ( 'NONE', *, *, #12927, .T. ) ;
#7962=CARTESIAN_POINT ( 'NONE',  ( -1.154700538379222596, 0.000000000000000000, -34.00000000000000000 ) ) ;
#7967=CARTESIAN_POINT ( 'NONE',  ( 47.32050807568875683, -37.00000000000000711, 41.96152422706633445 ) ) ;
#7972=CARTESIAN_POINT ( 'NONE',  ( -55.00000000000000000, 0.000000000000000000, 19.99999999999999289 ) ) ;
#7977=PLANE ( 'NONE',  #7220 ) ;
#7982=VECTOR ( 'NONE', #7564, 1000.000000000000114 ) ;
#7983=VECTOR ( 'NONE', #2398, 1000.000000000000000 ) ;
#7985=AXIS2_PLACEMENT_3D ( 'NONE', #10869, #8464, #7403 ) ;
#7991=CARTESIAN_POINT ( 'NONE',  ( 31.75426480542940766, -37.00000000000000711, 15.00000000000001243 ) ) ;
#7993=CARTESIAN_POINT ( 'NONE',  ( -44.43375672972994295, 0.000000000000000000, -19.99999999999594635 ) ) ;
#8002=EDGE_CURVE ( 'NONE', #15369, #8388, #1321, .T. ) ;
#8005=LINE ( 'NONE', #11688, #6098 ) ;
#8006=ORIENTED_EDGE ( 'NONE', *, *, #11241, .T. ) ;
#8017=VERTEX_POINT ( 'NONE', #3982 ) ;
#8030=CARTESIAN_POINT ( 'NONE',  ( 42.02221399786069611, -3.000000000000000000, -2.649999999999888445 ) ) ;
#8042=DIRECTION ( 'NONE',  ( 0.000000000000000000, -1.000000000000000000, 0.000000000000000000 ) ) ;
#8057=CARTESIAN_POINT ( 'NONE',  ( 42.02221399786069611, -3.000000000000001332, -2.649999999999881783 ) ) ;
#8083=CYLINDRICAL_SURFACE ( 'NONE', #5322, 32.00000000000000711 ) ;
#8084=LINE ( 'NONE', #5569, #9774 ) ;
#8088=CARTESIAN_POINT ( 'NONE',  ( -28.86751345948129455, -4.999999999999997335, 20.00000000000000355 ) ) ;
#8089=ADVANCED_FACE ( 'NONE', ( #823 ), #4616, .F. ) ;
#8092=FACE_OUTER_BOUND ( 'NONE', #1832, .T. ) ;
#8103=CYLINDRICAL_SURFACE ( 'NONE', #5822, 1.999999999999998668 ) ;
#8114=EDGE_LOOP ( 'NONE', ( #8789, #1542, #2184, #10939, #9742, #1869, #8754 ) ) ;
#8118=VERTEX_POINT ( 'NONE', #1862 ) ;
#8121=EDGE_CURVE ( 'NONE', #7289, #11317, #754, .T. ) ;
#8147=CARTESIAN_POINT ( 'NONE',  ( -13.27905619136138959, -35.00000000000000000, -59.00000000000000000 ) ) ;
#8149=DIRECTION ( 'NONE',  ( -1.734723475976807686E-15, 0.000000000000000000, 1.000000000000000000 ) ) ;
#8172=AXIS2_PLACEMENT_3D ( 'NONE', #2478, #15770, #7276 ) ;
#8174=CIRCLE ( 'NONE', #7902, 5.000000000000001776 ) ;
#8189=CARTESIAN_POINT ( 'NONE',  ( -4.618802153516124775, -3.000000000000000000, -36.00000000000148503 ) ) ;
#8193=CARTESIAN_POINT ( 'NONE',  ( -28.86751345948126257, -37.00000000000000711, -50.00000000000000711 ) ) ;
#8211=DIRECTION ( 'NONE',  ( -0.000000000000000000, -1.000000000000000000, -0.000000000000000000 ) ) ;
#8228=DIRECTION ( 'NONE',  ( -0.000000000000000000, 1.000000000000000000, -0.000000000000000000 ) ) ;
#8229=VECTOR ( 'NONE', #3597, 1000.000000000000000 ) ;
#8230=DIRECTION ( 'NONE',  ( 0.000000000000000000, -1.000000000000000000, 0.000000000000000000 ) ) ;
#8234=CARTESIAN_POINT ( 'NONE',  ( -28.86751345948126257, -35.00000000000000000, -50.00000000000000711 ) ) ;
#8246=PRODUCT_DEFINITION_SHAPE ( 'NONE', 'NONE',  #15797 ) ;
#8249=VECTOR ( 'NONE', #7886, 1000.000000000000000 ) ;
#8260=LINE ( 'NONE', #11932, #12052 ) ;
#8265=VERTEX_POINT ( 'NONE', #3470 ) ;
#8277=LINE ( 'NONE', #10761, #4693 ) ;
#8300=ORIENTED_EDGE ( 'NONE', *, *, #6079, .T. ) ;
#8305=EDGE_CURVE ( 'NONE', #2479, #6940, #13470, .T. ) ;
#8311=LINE ( 'NONE', #13201, #1231 ) ;
#8319=ORIENTED_EDGE ( 'NONE', *, *, #13016, .F. ) ;
#8324=DIRECTION ( 'NONE',  ( 0.8660254037844384856, 0.000000000000000000, -0.5000000000000004441 ) ) ;
#8334=CARTESIAN_POINT ( 'NONE',  ( -60.00000000000000000, -37.00000000000000711, 19.99999999999999289 ) ) ;
#8339=DIRECTION ( 'NONE',  ( 0.000000000000000000, 0.000000000000000000, 1.000000000000000000 ) ) ;
#8340=ORIENTED_EDGE ( 'NONE', *, *, #4679, .F. ) ;
#8370=CARTESIAN_POINT ( 'NONE',  ( -60.00000000000000000, -37.00000000000000711, 19.99999999999999289 ) ) ;
#8378=DIRECTION ( 'NONE',  ( 1.000000000000000000, 0.000000000000000000, 1.114413700119375779E-16 ) ) ;
#8384=DIRECTION ( 'NONE',  ( 0.000000000000000000, 0.000000000000000000, 1.000000000000000000 ) ) ;
#8388=VERTEX_POINT ( 'NONE', #1536 ) ;
#8390=ORIENTED_EDGE ( 'NONE', *, *, #3783, .F. ) ;
#8394=CARTESIAN_POINT ( 'NONE',  ( -2.886751345948099789, -37.00000000000000711, -35.00000000000000000 ) ) ;
#8404=LINE ( 'NONE', #13296, #4067 ) ;
#8409=ORIENTED_EDGE ( 'NONE', *, *, #1571, .T. ) ;
#8428=AXIS2_PLACEMENT_3D ( 'NONE', #15925, #9849, #15772 ) ;
#8436=CARTESIAN_POINT ( 'NONE',  ( 42.02221399786069611, 0.000000000000000000, 2.650000000000096723 ) ) ;
#8464=DIRECTION ( 'NONE',  ( -0.8660254037844389297, -0.000000000000000000, 0.4999999999999997780 ) ) ;
#8469=CARTESIAN_POINT ( 'NONE',  ( -28.86751345948126257, -37.00000000000000711, -50.00000000000000711 ) ) ;
#8483=AXIS2_PLACEMENT_3D ( 'NONE', #4254, #14119, #3046 ) ;
#8486=EDGE_CURVE ( 'NONE', #11087, #15683, #3147, .T. ) ;
#8488=AXIS2_PLACEMENT_3D ( 'NONE', #14898, #5115, #11167 ) ;
#8514=LINE ( 'NONE', #984, #14648 ) ;
#8549=DIRECTION ( 'NONE',  ( 0.4999999999999998335, 0.000000000000000000, 0.8660254037844387076 ) ) ;
#8562=LINE ( 'NONE', #8637, #2009 ) ;
#8565=ORIENTED_EDGE ( 'NONE', *, *, #13908, .F. ) ;
#8571=CARTESIAN_POINT ( 'NONE',  ( -28.86751345948128744, -35.00000000000000000, 17.99999999999999645 ) ) ;
#8574=EDGE_CURVE ( 'NONE', #12974, #5996, #8260, .T. ) ;
#8575=EDGE_CURVE ( 'NONE', #15092, #8265, #9246, .T. ) ;
#8578=DIRECTION ( 'NONE',  ( 0.000000000000000000, 0.000000000000000000, 1.000000000000000000 ) ) ;
#8580=CARTESIAN_POINT ( 'NONE',  ( -2.886751345948130432, -5.000000000000000000, 35.00000000000001421 ) ) ;
#8587=ORIENTED_EDGE ( 'NONE', *, *, #63, .T. ) ;
#8599=CARTESIAN_POINT ( 'NONE',  ( -21.01110699893060030, 0.000000000000000000, 33.74230484541324415 ) ) ;
#8604=EDGE_LOOP ( 'NONE', ( #7705, #12102, #827, #2961 ) ) ;
#8622=FACE_OUTER_BOUND ( 'NONE', #12232, .T. ) ;
#8634=DIRECTION ( 'NONE',  ( -1.000000000000000000, -0.000000000000000000, -3.343241100358131282E-16 ) ) ;
#8637=CARTESIAN_POINT ( 'NONE',  ( 31.75426480542940766, -37.00000000000000711, 15.00000000000001066 ) ) ;
#8643=VERTEX_POINT ( 'NONE', #4592 ) ;
#8650=DIRECTION ( 'NONE',  ( -0.5000000000000002220, 0.000000000000000000, 0.8660254037844383745 ) ) ;
#8651=DIRECTION ( 'NONE',  ( 0.000000000000000000, 0.000000000000000000, 1.000000000000000000 ) ) ;
#8653=DIRECTION ( 'NONE',  ( 0.000000000000000000, -1.000000000000000000, 0.000000000000000000 ) ) ;
#8677=DIRECTION ( 'NONE',  ( 0.4999999999999998335, -0.000000000000000000, 0.8660254037844387076 ) ) ;
#8681=DIRECTION ( 'NONE',  ( 0.000000000000000000, 0.000000000000000000, 1.000000000000000000 ) ) ;
#8697=DIRECTION ( 'NONE',  ( -0.000000000000000000, 1.000000000000000000, -0.000000000000000000 ) ) ;
#8708=ORIENTED_EDGE ( 'NONE', *, *, #3445, .F. ) ;
#8711=DIRECTION ( 'NONE',  ( -0.8660254037844387076, 0.000000000000000000, 0.4999999999999997224 ) ) ;
#8718=EDGE_CURVE ( 'NONE', #3403, #14772, #5969, .T. ) ;
#8722=EDGE_CURVE ( 'NONE', #11884, #11709, #8562, .T. ) ;
#8733=VECTOR ( 'NONE', #15639, 1000.000000000000000 ) ;
#8734=FACE_OUTER_BOUND ( 'NONE', #12454, .T. ) ;
#8753=VECTOR ( 'NONE', #9176, 1000.000000000000114 ) ;
#8754=ORIENTED_EDGE ( 'NONE', *, *, #13922, .F. ) ;
#8773=EDGE_CURVE ( 'NONE', #3387, #7945, #8404, .T. ) ;
#8775=B_SPLINE_CURVE_WITH_KNOTS ( 'NONE', 3,
 ( #4278, #10423, #3952, #12667, #13800, #4116, #9064, #5420, #14141, #2737, #11622, #15358, #1535, #7693, #15279, #2822 ),
 .UNSPECIFIED., .F., .F.,
 ( 4, 2, 2, 2, 2, 2, 2, 4 ),
 ( 0.000000000000000000, 0.0003988081628697498124, 0.0007976163257394996249, 0.001196424488609249383, 0.001595232651478999250, 0.001994040814348749333, 0.002392848977218498766, 0.003190465302957996331 ),
 .UNSPECIFIED. ) ;
#8789=ORIENTED_EDGE ( 'NONE', *, *, #10275, .T. ) ;
#8802=EDGE_LOOP ( 'NONE', ( #6517, #5974 ) ) ;
#8831=CARTESIAN_POINT ( 'NONE',  ( -28.86751345948129455, -3.000000000000000000, 22.00000000000000711 ) ) ;
#8853=CARTESIAN_POINT ( 'NONE',  ( 14.41154273188009682, -35.00000000000000000, 60.96152422706633445 ) ) ;
#8903=( NAMED_UNIT ( * ) SI_UNIT ( $, .STERADIAN. ) SOLID_ANGLE_UNIT ( ) );
#8907=EDGE_CURVE ( 'NONE', #6536, #7472, #5230, .T. ) ;
#8911=CARTESIAN_POINT ( 'NONE',  ( -44.43024643319441225, -4.732646668676770751, 20.01350297727719507 ) ) ;
#8916=AXIS2_PLACEMENT_3D ( 'NONE', #9274, #855, #626 ) ;
#8941=ORIENTED_EDGE ( 'NONE', *, *, #8575, .T. ) ;
#8942=DIRECTION ( 'NONE',  ( 0.5000000000000002220, 0.000000000000000000, -0.8660254037844384856 ) ) ;
#8946=ORIENTED_EDGE ( 'NONE', *, *, #13380, .F. ) ;
#8971=ORIENTED_EDGE ( 'NONE', *, *, #10175, .F. ) ;
#8974=DIRECTION ( 'NONE',  ( 1.114413700119375779E-16, 0.000000000000000000, -1.000000000000000000 ) ) ;
#8988=ORIENTED_EDGE ( 'NONE', *, *, #4725, .F. ) ;
#8989=ORIENTED_EDGE ( 'NONE', *, *, #15462, .F. ) ;
#8992=DIRECTION ( 'NONE',  ( 0.000000000000000000, 0.000000000000000000, 1.000000000000000000 ) ) ;
#8994=CYLINDRICAL_SURFACE ( 'NONE', #4315, 4.999999999999997335 ) ;
#9006=CARTESIAN_POINT ( 'NONE',  ( 2.875844205641825191, -3.000000000000000000, -48.98110827882413787 ) ) ;
#9008=FILL_AREA_STYLE ('',( #5120 ) ) ;
#9012=CIRCLE ( 'NONE', #14950, 2.649999999999992806 ) ;
#9014=ORIENTED_EDGE ( 'NONE', *, *, #12842, .T. ) ;
#9019=VECTOR ( 'NONE', #9212, 1000.000000000000000 ) ;
#9020=EDGE_CURVE ( 'NONE', #7038, #12621, #5370, .T. ) ;
#9031=CARTESIAN_POINT ( 'NONE',  ( -60.00000000000000000, -5.000000000000000000, 17.99999999999999289 ) ) ;
#9061=CARTESIAN_POINT ( 'NONE',  ( -21.01110699893041911, -3.000000000000000000, -36.39230484541334221 ) ) ;
#9064=CARTESIAN_POINT ( 'NONE',  ( -44.15480264658854992, -3.253774389711709958, -21.01641944516413574 ) ) ;
#9069=ADVANCED_FACE ( 'NONE', ( #10335 ), #15340, .T. ) ;
#9071=VERTEX_POINT ( 'NONE', #7993 ) ;
#9080=DIRECTION ( 'NONE',  ( -0.000000000000000000, -1.000000000000000000, -0.000000000000000000 ) ) ;
#9084=EDGE_LOOP ( 'NONE', ( #13709, #14657, #15858, #4039, #12773 ) ) ;
#9087=CARTESIAN_POINT ( 'NONE',  ( -28.86751345948130165, 0.000000000000000000, 18.00000000000000355 ) ) ;
#9101=FACE_OUTER_BOUND ( 'NONE', #9084, .T. ) ;
#9104=VERTEX_POINT ( 'NONE', #3507 ) ;
#9105=DIRECTION ( 'NONE',  ( 0.5000000000000002220, 2.602085213965209853E-15, -0.8660254037844383745 ) ) ;
#9131=ORIENTED_EDGE ( 'NONE', *, *, #15493, .T. ) ;
#9132=VECTOR ( 'NONE', #11231, 1000.000000000000114 ) ;
#9150=DIRECTION ( 'NONE',  ( 1.000000000000000000, 0.000000000000000000, 1.114413700119375779E-16 ) ) ;
#9157=CARTESIAN_POINT ( 'NONE',  ( -21.01110699893041911, -3.000000000000000000, -33.74230484541335073 ) ) ;
#9166=ORIENTED_EDGE ( 'NONE', *, *, #9463, .F. ) ;
#9176=DIRECTION ( 'NONE',  ( 0.8660254037844383745, -0.000000000000000000, 0.5000000000000004441 ) ) ;
#9199=DIRECTION ( 'NONE',  ( 0.8660254037844383745, 0.000000000000000000, 0.5000000000000004441 ) ) ;
#9204=VECTOR ( 'NONE', #866, 1000.000000000000000 ) ;
#9205=CARTESIAN_POINT ( 'NONE',  ( 44.82050807568879947, 0.000000000000000000, -37.63139720814411504 ) ) ;
#9206=ORIENTED_EDGE ( 'NONE', *, *, #14897, .T. ) ;
#9212=DIRECTION ( 'NONE',  ( -0.000000000000000000, 1.000000000000000000, -0.000000000000000000 ) ) ;
#9222=ORIENTED_EDGE ( 'NONE', *, *, #1950, .T. ) ;
#9229=CARTESIAN_POINT ( 'NONE',  ( -43.89750408695873318, -2.999999999999999112, 21.87156796334076247 ) ) ;
#9236=ADVANCED_FACE ( 'NONE', ( #11350 ), #9893, .T. ) ;
#9246=CIRCLE ( 'NONE', #11295, 2.649999999999992806 ) ;
#9264=LINE ( 'NONE', #7972, #12538 ) ;
#9266=CARTESIAN_POINT ( 'NONE',  ( 12.67949192431120586, -37.00000000000000711, 61.96152422706632024 ) ) ;
#9269=EDGE_CURVE ( 'NONE', #11087, #7869, #3987, .T. ) ;
#9274=CARTESIAN_POINT ( 'NONE',  ( 10.17949192431126448, -5.000000000000000000, -57.63139720814413636 ) ) ;
#9279=CARTESIAN_POINT ( 'NONE',  ( -16.18981371719892692, -5.000000000000000000, 15.95842007673591745 ) ) ;
#9308=EDGE_LOOP ( 'NONE', ( #14595, #12897, #3588, #9565 ) ) ;
#9310=EDGE_CURVE ( 'NONE', #11317, #9517, #5689, .T. ) ;
#9316=CARTESIAN_POINT ( 'NONE',  ( 39.53738644055469820, -5.000000000000000000, -28.48076211352550047 ) ) ;
#9328=CARTESIAN_POINT ( 'NONE',  ( 39.61557500986572933, -4.342938577511704423, 28.40349439876419169 ) ) ;
#9348=FACE_OUTER_BOUND ( 'NONE', #13787, .T. ) ;
#9350=DIRECTION ( 'NONE',  ( -0.4999999999999997780, -0.000000000000000000, -0.8660254037844389297 ) ) ;
#9377=ORIENTED_EDGE ( 'NONE', *, *, #3298, .F. ) ;
#9379=CARTESIAN_POINT ( 'NONE',  ( -4.618802153516976539, -4.999999999999997335, -36.00000000000000711 ) ) ;
#9382=LINE ( 'NONE', #6729, #512 ) ;
#9386=DIRECTION ( 'NONE',  ( -0.000000000000000000, -1.000000000000000000, -0.000000000000000000 ) ) ;
#9387=LINE ( 'NONE', #14310, #12444 ) ;
#9389=LINE ( 'NONE', #8189, #4172 ) ;
#9399=LINE ( 'NONE', #15547, #11086 ) ;
#9400=VERTEX_POINT ( 'NONE', #10781 ) ;
#9404=CARTESIAN_POINT ( 'NONE',  ( 14.41154273188013590, -5.000000000000004441, -60.96152422706631313 ) ) ;
#9409=CARTESIAN_POINT ( 'NONE',  ( -21.01110699893060030, -3.000000000000000000, 33.74230484541324415 ) ) ;
#9419=ORIENTED_EDGE ( 'NONE', *, *, #11853, .T. ) ;
#9427=CARTESIAN_POINT ( 'NONE',  ( 47.32050807568879947, -37.00000000000000711, -41.96152422706630603 ) ) ;
#9428=DIRECTION ( 'NONE',  ( -0.8660254037844385966, 0.000000000000000000, 0.5000000000000000000 ) ) ;
#9438=AXIS2_PLACEMENT_3D ( 'NONE', #11153, #7532, #12434 ) ;
#9441=FACE_OUTER_BOUND ( 'NONE', #135, .T. ) ;
#9454=DIRECTION ( 'NONE',  ( -0.000000000000000000, 1.000000000000000000, -0.000000000000000000 ) ) ;
#9455=ORIENTED_EDGE ( 'NONE', *, *, #102, .F. ) ;
#9462=EDGE_CURVE ( 'NONE', #12753, #1232, #5388, .T. ) ;
#9463=EDGE_CURVE ( 'NONE', #5239, #10374, #12857, .T. ) ;
#9470=DIRECTION ( 'NONE',  ( -1.000000000000000000, 0.000000000000000000, -3.343241100358131282E-16 ) ) ;
#9476=DIRECTION ( 'NONE',  ( 0.8660254037844387076, 0.000000000000000000, -0.4999999999999997224 ) ) ;
#9502=ADVANCED_FACE ( 'NONE', ( #6416 ), #13741, .T. ) ;
#9505=CARTESIAN_POINT ( 'NONE',  ( 47.32050807568875683, -37.00000000000000711, 41.96152422706633445 ) ) ;
#9515=ORIENTED_EDGE ( 'NONE', *, *, #7862, .F. ) ;
#9517=VERTEX_POINT ( 'NONE', #12528 ) ;
#9524=DIRECTION ( 'NONE',  ( 0.5000000000000003331, -6.505213034913029562E-16, 0.8660254037844385966 ) ) ;
#9542=LINE ( 'NONE', #5818, #6057 ) ;
#9548=DIRECTION ( 'NONE',  ( -1.000000000000000000, 2.602085213965212219E-15, 0.000000000000000000 ) ) ;
#9549=FACE_OUTER_BOUND ( 'NONE', #6539, .T. ) ;
#9551=EDGE_CURVE ( 'NONE', #1675, #2479, #11334, .T. ) ;
#9565=ORIENTED_EDGE ( 'NONE', *, *, #1278, .T. ) ;
#9571=CARTESIAN_POINT ( 'NONE',  ( 30.02221399786052913, 88.59290746114278647, 16.00000000000001066 ) ) ;
#9591=DIRECTION ( 'NONE',  ( -0.000000000000000000, 1.000000000000000000, -0.000000000000000000 ) ) ;
#9603=CARTESIAN_POINT ( 'NONE',  ( 42.02221399786069611, 0.000000000000000000, 1.040834085586084257E-13 ) ) ;
#9615=CARTESIAN_POINT ( 'NONE',  ( -28.86751345948130165, -37.00000000000000711, 20.00000000000000355 ) ) ;
#9623=EDGE_LOOP ( 'NONE', ( #159, #1813, #12038, #5786 ) ) ;
#9642=DIRECTION ( 'NONE',  ( -0.4999999999999997780, 0.000000000000000000, -0.8660254037844388186 ) ) ;
#9647=CARTESIAN_POINT ( 'NONE',  ( -28.86751345948130165, 88.59290746114278647, 18.00000000000000355 ) ) ;
#9654=ORIENTED_EDGE ( 'NONE', *, *, #6405, .F. ) ;
#9659=DIRECTION ( 'NONE',  ( -0.4999999999999997224, 0.000000000000000000, -0.8660254037844388186 ) ) ;
#9664=EDGE_CURVE ( 'NONE', #7472, #2457, #6164, .T. ) ;
#9666=DIRECTION ( 'NONE',  ( -0.000000000000000000, 1.000000000000000000, -0.000000000000000000 ) ) ;
#9691=AXIS2_PLACEMENT_3D ( 'NONE', #3232, #15688, #14154 ) ;
#9697=DIRECTION ( 'NONE',  ( 0.000000000000000000, 0.000000000000000000, -1.000000000000000000 ) ) ;
#9704=FACE_OUTER_BOUND ( 'NONE', #10724, .T. ) ;
#9722=FACE_OUTER_BOUND ( 'NONE', #14124, .T. ) ;
#9738=VECTOR ( 'NONE', #11272, 1000.000000000000000 ) ;
#9742=ORIENTED_EDGE ( 'NONE', *, *, #2412, .T. ) ;
#9753=DIRECTION ( 'NONE',  ( -4.336808689942013792E-16, 0.000000000000000000, 1.000000000000000000 ) ) ;
#9771=ORIENTED_EDGE ( 'NONE', *, *, #3162, .F. ) ;
#9773=AXIS2_PLACEMENT_3D ( 'NONE', #3163, #13242, #9548 ) ;
#9774=VECTOR ( 'NONE', #6626, 1000.000000000000000 ) ;
#9779=CARTESIAN_POINT ( 'NONE',  ( -44.43375672972994295, -3.000000000000000000, -22.00000000000000355 ) ) ;
#9782=DIRECTION ( 'NONE',  ( 0.8660254037844387076, 0.000000000000000000, -0.4999999999999997224 ) ) ;
#9833=ADVANCED_FACE ( 'NONE', ( #7601, #6228 ), #12498, .F. ) ;
#9849=DIRECTION ( 'NONE',  ( 0.8660254037844385966, 0.000000000000000000, 0.5000000000000003331 ) ) ;
#9860=LINE ( 'NONE', #13649, #2914 ) ;
#9862=SURFACE_SIDE_STYLE ('',( #2660 ) ) ;
#9870=ADVANCED_FACE ( 'NONE', ( #15104 ), #9928, .F. ) ;
#9893=CYLINDRICAL_SURFACE ( 'NONE', #2272, 40.00000000000000711 ) ;
#9899=EDGE_LOOP ( 'NONE', ( #11472, #4900, #11379, #659, #10076, #12380, #13566 ) ) ;
#9903=FACE_OUTER_BOUND ( 'NONE', #6897, .T. ) ;
#9907=DIRECTION ( 'NONE',  ( -1.000000000000000000, -1.734723475976808080E-15, 0.000000000000000000 ) ) ;
#9916=DIRECTION ( 'NONE',  ( 0.000000000000000000, 0.000000000000000000, -1.000000000000000000 ) ) ;
#9928=PLANE ( 'NONE',  #6429 ) ;
#9945=EDGE_CURVE ( 'NONE', #11703, #1559, #10347, .T. ) ;
#9951=CARTESIAN_POINT ( 'NONE',  ( 39.90939079054413696, -3.661800705854930893, 28.10922023582534379 ) ) ;
#9954=VECTOR ( 'NONE', #6297, 1000.000000000000114 ) ;
#9959=VECTOR ( 'NONE', #1336, 1000.000000000000000 ) ;
#9963=DIRECTION ( 'NONE',  ( -1.000000000000000000, 0.000000000000000000, -3.343241100358131282E-16 ) ) ;
#9965=EDGE_CURVE ( 'NONE', #1559, #4540, #7925, .T. ) ;
#9985=EDGE_CURVE ( 'NONE', #6711, #3387, #8084, .T. ) ;
#9987=ORIENTED_EDGE ( 'NONE', *, *, #9269, .T. ) ;
#9994=AXIS2_PLACEMENT_3D ( 'NONE', #287, #1479, #5275 ) ;
#10009=ORIENTED_EDGE ( 'NONE', *, *, #12929, .T. ) ;
#10010=DIRECTION ( 'NONE',  ( -0.8660254037844383745, -0.000000000000000000, -0.5000000000000005551 ) ) ;
#10020=DIRECTION ( 'NONE',  ( -1.000000000000000000, 0.000000000000000000, -1.114413700119375779E-16 ) ) ;
#10030=DIRECTION ( 'NONE',  ( -0.000000000000000000, 1.000000000000000000, -0.000000000000000000 ) ) ;
#10036=VERTEX_POINT ( 'NONE', #3064 ) ;
#10056=LINE ( 'NONE', #10131, #1191 ) ;
#10063=DIRECTION ( 'NONE',  ( -0.8660254037844385966, 0.000000000000000000, -0.5000000000000002220 ) ) ;
#10076=ORIENTED_EDGE ( 'NONE', *, *, #12141, .T. ) ;
#10083=EDGE_CURVE ( 'NONE', #10415, #8643, #9382, .T. ) ;
#10087=FACE_OUTER_BOUND ( 'NONE', #526, .T. ) ;
#10113=VERTEX_POINT ( 'NONE', #15529 ) ;
#10116=DIRECTION ( 'NONE',  ( -0.4999999999999997224, 0.000000000000000000, -0.8660254037844388186 ) ) ;
#10128=( NAMED_UNIT ( * ) PLANE_ANGLE_UNIT ( ) SI_UNIT ( $, .RADIAN. ) );
#10131=CARTESIAN_POINT ( 'NONE',  ( 12.67949192431120764, -5.000000000000000000, 61.96152422706632024 ) ) ;
#10138=AXIS2_PLACEMENT_3D ( 'NONE', #1101, #8634, #9753 ) ;
#10147=ORIENTED_EDGE ( 'NONE', *, *, #8486, .T. ) ;
#10159=DIRECTION ( 'NONE',  ( 0.000000000000000000, -1.000000000000000000, 0.000000000000000000 ) ) ;
#10169=ORIENTED_EDGE ( 'NONE', *, *, #8907, .T. ) ;
#10175=EDGE_CURVE ( 'NONE', #12753, #7038, #10671, .T. ) ;
#10177=EDGE_CURVE ( 'NONE', #5996, #7857, #11579, .T. ) ;
#10184=DIRECTION ( 'NONE',  ( 0.000000000000000000, 0.000000000000000000, -1.000000000000000000 ) ) ;
#10193=ORIENTED_EDGE ( 'NONE', *, *, #11128, .F. ) ;
#10195=VECTOR ( 'NONE', #10959, 1000.000000000000114 ) ;
#10204=AXIS2_PLACEMENT_3D ( 'NONE', #10243, #10159, #465 ) ;
#10209=CARTESIAN_POINT ( 'NONE',  ( 40.98096197215471648, -3.000000000000000000, -26.98110827881998119 ) ) ;
#10211=MECHANICAL_DESIGN_GEOMETRIC_PRESENTATION_REPRESENTATION('',(#13021),#10972);
#10212=CARTESIAN_POINT ( 'NONE',  ( 4.388603409518465170, -3.661800705854443727, -48.61715639207540107 ) ) ;
#10224=AXIS2_PLACEMENT_3D ( 'NONE', #7351, #12105, #8339 ) ;
#10241=DIRECTION ( 'NONE',  ( 0.000000000000000000, -0.000000000000000000, -1.000000000000000000 ) ) ;
#10242=VECTOR ( 'NONE', #1436, 1000.000000000000114 ) ;
#10243=CARTESIAN_POINT ( 'NONE',  ( -28.86751345948126257, -3.000000000000000000, -50.00000000000000711 ) ) ;
#10268=DIRECTION ( 'NONE',  ( -0.000000000000000000, 1.000000000000000000, 0.000000000000000000 ) ) ;
#10275=EDGE_CURVE ( 'NONE', #621, #14429, #5896, .T. ) ;
#10295=EDGE_CURVE ( 'NONE', #11118, #4347, #12080, .T. ) ;
#10313=UNCERTAINTY_MEASURE_WITH_UNIT (LENGTH_MEASURE( 1.000000000000000082E-05 ), #5272, 'distance_accuracy_value', 'NONE');
#10332=LINE ( 'NONE', #4168, #11830 ) ;
#10335=FACE_OUTER_BOUND ( 'NONE', #12688, .T. ) ;
#10347=LINE ( 'NONE', #15274, #9019 ) ;
#10362=ORIENTED_EDGE ( 'NONE', *, *, #9551, .T. ) ;
#10364=ADVANCED_FACE ( 'NONE', ( #13633 ), #7977, .F. ) ;
#10374=VERTEX_POINT ( 'NONE', #161 ) ;
#10384=DIRECTION ( 'NONE',  ( -0.5000000000000005551, 0.000000000000000000, 0.8660254037844382635 ) ) ;
#10385=DIRECTION ( 'NONE',  ( 0.000000000000000000, 0.000000000000000000, -1.000000000000000000 ) ) ;
#10389=CARTESIAN_POINT ( 'NONE',  ( 30.02221399786053979, -35.00000000000000000, -15.99999999999998579 ) ) ;
#10390=ORIENTED_EDGE ( 'NONE', *, *, #183, .F. ) ;
#10392=ORIENTED_EDGE ( 'NONE', *, *, #15255, .F. ) ;
#10397=EDGE_CURVE ( 'NONE', #6220, #11087, #6713, .T. ) ;
#10400=CYLINDRICAL_SURFACE ( 'NONE', #347, 40.00000000000001421 ) ;
#10415=VERTEX_POINT ( 'NONE', #15404 ) ;
#10423=CARTESIAN_POINT ( 'NONE',  ( -43.89752705808261624, -2.999999999999999556, -21.87149547239932090 ) ) ;
#10432=CIRCLE ( 'NONE', #3444, 2.000000000000001776 ) ;
#10436=ORIENTED_EDGE ( 'NONE', *, *, #2079, .F. ) ;
#10450=ORIENTED_EDGE ( 'NONE', *, *, #2365, .T. ) ;
#10451=CARTESIAN_POINT ( 'NONE',  ( 31.75426480542940766, 0.000000000000000000, 15.00000000000001066 ) ) ;
#10455=CIRCLE ( 'NONE', #10204, 28.00000000000000355 ) ;
#10472=CARTESIAN_POINT ( 'NONE',  ( 43.08845726811992449, -5.000000000000000000, -38.63139720814411504 ) ) ;
#10484=CYLINDRICAL_SURFACE ( 'NONE', #13864, 2.000000000000001776 ) ;
#10497=EDGE_LOOP ( 'NONE', ( #5427, #7042, #11393, #11133 ) ) ;
#10503=LINE ( 'NONE', #15515, #13817 ) ;
#10504=AXIS2_PLACEMENT_3D ( 'NONE', #3188, #1810, #5693 ) ;
#10510=CLOSED_SHELL ( 'NONE', ( #15160, #2643, #1345, #12931, #7187, #11149, #13015, #7540, #15670, #10364, #14424, #15472, #10608, #11147, #12206, #14486, #3236, #13570, #5630, #1509, #11814, #6096, #2384, #9870, #7685, #4962, #7922, #10666, #13304, #4844, #2663, #1895, #4069, #1859, #9833, #9236, #11283, #15862, #8089, #1842, #4336, #11506, #5379, #1839, #1681, #12047, #519, #9502, #9069, #381, #12720, #14031, #10736, #13076 ) ) ;
#10527=CARTESIAN_POINT ( 'NONE',  ( 40.12140847263850674, -3.395032785697077671, -27.89299687554618856 ) ) ;
#10539=AXIS2_PLACEMENT_3D ( 'NONE', #4710, #13664, #5358 ) ;
#10547=CARTESIAN_POINT ( 'NONE',  ( 39.58615490320391217, -4.472255266398825313, 28.43259952176492433 ) ) ;
#10551=PRODUCT ( 'Precision Linear Jaw Guides', 'Precision Linear Jaw Guides', '', ( #5676 ) ) ;
#10555=LINE ( 'NONE', #9409, #3225 ) ;
#10581=VERTEX_POINT ( 'NONE', #8057 ) ;
#10583=DIRECTION ( 'NONE',  ( -0.000000000000000000, 1.000000000000000000, -0.000000000000000000 ) ) ;
#10594=CARTESIAN_POINT ( 'NONE',  ( 3.391751934957232706, -3.060691311048527652, 48.86415051386519082 ) ) ;
#10598=CARTESIAN_POINT ( 'NONE',  ( 45.58845726811992449, 88.59290746114278647, -42.96152422706630603 ) ) ;
#10608=ADVANCED_FACE ( 'NONE', ( #9722 ), #2291, .F. ) ;
#10621=CARTESIAN_POINT ( 'NONE',  ( 39.53738644056090124, -5.000000000000000000, 28.48076211354432985 ) ) ;
#10641=DIRECTION ( 'NONE',  ( 1.000000000000000000, 0.000000000000000000, 1.114413700119375779E-16 ) ) ;
#10649=EDGE_CURVE ( 'NONE', #13587, #10806, #2601, .T. ) ;
#10651=ORIENTED_EDGE ( 'NONE', *, *, #1574, .F. ) ;
#10666=ADVANCED_FACE ( 'NONE', ( #202 ), #15958, .F. ) ;
#10669=EDGE_LOOP ( 'NONE', ( #7470, #4074, #487, #7661, #13979, #181 ) ) ;
#10671=LINE ( 'NONE', #4202, #14943 ) ;
#10683=DIRECTION ( 'NONE',  ( 3.343241100358131282E-16, 0.000000000000000000, -1.000000000000000000 ) ) ;
#10685=VERTEX_POINT ( 'NONE', #12293 ) ;
#10691=CARTESIAN_POINT ( 'NONE',  ( -5.725490332117410652, 0.000000000000000000, 49.91684015347181003 ) ) ;
#10694=CARTESIAN_POINT ( 'NONE',  ( 11.91154273188008439, 0.000000000000000000, 56.63139720814412925 ) ) ;
#10711=DIRECTION ( 'NONE',  ( 0.4999999999999998335, -0.000000000000000000, 0.8660254037844387076 ) ) ;
#10718=AXIS2_PLACEMENT_3D ( 'NONE', #13590, #11176, #118 ) ;
#10724=EDGE_LOOP ( 'NONE', ( #4578, #543, #11682, #4516 ) ) ;
#10736=ADVANCED_FACE ( 'NONE', ( #14081 ), #12533, .F. ) ;
#10746=DIRECTION ( 'NONE',  ( 0.8660254037844384856, 0.000000000000000000, 0.5000000000000004441 ) ) ;
#10747=VERTEX_POINT ( 'NONE', #6571 ) ;
#10761=CARTESIAN_POINT ( 'NONE',  ( -28.86751345948126612, -35.00000000000000000, -18.00000000000000355 ) ) ;
#10763=DIRECTION ( 'NONE',  ( 0.4999999999999998890, 0.000000000000000000, 0.8660254037844388186 ) ) ;
#10768=ORIENTED_EDGE ( 'NONE', *, *, #7153, .F. ) ;
#10781=CARTESIAN_POINT ( 'NONE',  ( -60.00000000000000000, -35.00000000000000000, 17.99999999999999289 ) ) ;
#10783=LINE ( 'NONE', #10855, #14164 ) ;
#10794=AXIS2_PLACEMENT_3D ( 'NONE', #11645, #1715, #7799 ) ;
#10797=CARTESIAN_POINT ( 'NONE',  ( 41.26943724812357317, -3.000000000000000000, -27.48076211352550047 ) ) ;
#10798=CARTESIAN_POINT ( 'NONE',  ( 11.91154273188008084, -5.000000000000000000, 56.63139720814412925 ) ) ;
#10806=VERTEX_POINT ( 'NONE', #11410 ) ;
#10813=AXIS2_PLACEMENT_3D ( 'NONE', #5999, #7374, #6169 ) ;
#10826=EDGE_LOOP ( 'NONE', ( #2362, #6479, #14191, #11157, #13658 ) ) ;
#10853=DIRECTION ( 'NONE',  ( 0.8660254037844384856, 0.000000000000000000, 0.5000000000000001110 ) ) ;
#10854=ORIENTED_EDGE ( 'NONE', *, *, #3445, .T. ) ;
#10855=CARTESIAN_POINT ( 'NONE',  ( -44.45597072760116220, -35.00000000000000000, -41.00000000000001421 ) ) ;
#10856=EDGE_CURVE ( 'NONE', #5667, #1764, #12691, .T. ) ;
#10860=ORIENTED_EDGE ( 'NONE', *, *, #9310, .T. ) ;
#10861=EDGE_CURVE ( 'NONE', #4061, #15286, #435, .T. ) ;
#10869=CARTESIAN_POINT ( 'NONE',  ( 10.17949192431120586, -5.000000000000000000, 57.63139720814412215 ) ) ;
#10875=EDGE_CURVE ( 'NONE', #560, #15871, #9399, .T. ) ;
#10877=ORIENTED_EDGE ( 'NONE', *, *, #11555, .F. ) ;
#10879=EDGE_CURVE ( 'NONE', #395, #7055, #6901, .T. ) ;
#10884=DIRECTION ( 'NONE',  ( -0.000000000000000000, 1.000000000000000000, -0.000000000000000000 ) ) ;
#10890=DIRECTION ( 'NONE',  ( 0.000000000000000000, -1.000000000000000000, 0.000000000000000000 ) ) ;
#10894=DIRECTION ( 'NONE',  ( -0.5000000000000003331, -2.168404344971013059E-16, 0.8660254037844384856 ) ) ;
#10901=LINE ( 'NONE', #13393, #10242 ) ;
#10910=EDGE_CURVE ( 'NONE', #8643, #6940, #11959, .T. ) ;
#10921=ORIENTED_EDGE ( 'NONE', *, *, #6341, .T. ) ;
#10939=ORIENTED_EDGE ( 'NONE', *, *, #5000, .F. ) ;
#10946=DIRECTION ( 'NONE',  ( 0.8660254037844389297, -0.000000000000000000, -0.4999999999999997780 ) ) ;
#10953=CARTESIAN_POINT ( 'NONE',  ( -60.00000000000000000, -37.00000000000000711, 19.99999999999999289 ) ) ;
#10955=ORIENTED_EDGE ( 'NONE', *, *, #12598, .T. ) ;
#10959=DIRECTION ( 'NONE',  ( -0.5000000000000005551, -0.000000000000000000, 0.8660254037844382635 ) ) ;
#10972=( GEOMETRIC_REPRESENTATION_CONTEXT ( 3 ) GLOBAL_UNCERTAINTY_ASSIGNED_CONTEXT ( ( #10313 ) ) GLOBAL_UNIT_ASSIGNED_CONTEXT ( ( #5272, #11571, #15138 ) ) REPRESENTATION_CONTEXT ( 'NONE', 'WORKASPACE' ) );
#10979=ORIENTED_EDGE ( 'NONE', *, *, #9462, .T. ) ;
#10994=DIRECTION ( 'NONE',  ( -0.4999999999999997224, -0.000000000000000000, -0.8660254037844388186 ) ) ;
#11009=CIRCLE ( 'NONE', #10539, 5.000000000000001776 ) ;
#11022=ORIENTED_EDGE ( 'NONE', *, *, #6200, .F. ) ;
#11032=CARTESIAN_POINT ( 'NONE',  ( 12.67949192431126093, -4.999999999999997335, -61.96152422706632024 ) ) ;
#11040=DIRECTION ( 'NONE',  ( -0.8660254037844390407, 0.000000000000000000, 0.4999999999999993339 ) ) ;
#11052=LINE ( 'NONE', #13216, #6892 ) ;
#11069=DIRECTION ( 'NONE',  ( -1.000000000000000000, 0.000000000000000000, 0.000000000000000000 ) ) ;
#11085=ORIENTED_EDGE ( 'NONE', *, *, #3298, .T. ) ;
#11086=VECTOR ( 'NONE', #8042, 1000.000000000000000 ) ;
#11087=VERTEX_POINT ( 'NONE', #7539 ) ;
#11098=CARTESIAN_POINT ( 'NONE',  ( -28.86751345948130165, -37.00000000000000711, 20.00000000000000355 ) ) ;
#11099=ORIENTED_EDGE ( 'NONE', *, *, #2188, .F. ) ;
#11100=DIRECTION ( 'NONE',  ( -0.000000000000000000, 1.000000000000000000, -0.000000000000000000 ) ) ;
#11118=VERTEX_POINT ( 'NONE', #8436 ) ;
#11120=ORIENTED_EDGE ( 'NONE', *, *, #11812, .T. ) ;
#11128=EDGE_CURVE ( 'NONE', #13637, #2243, #15386, .T. ) ;
#11133=ORIENTED_EDGE ( 'NONE', *, *, #10879, .F. ) ;
#11137=DIRECTION ( 'NONE',  ( 0.8660254037844388186, 0.000000000000000000, -0.4999999999999997224 ) ) ;
#11140=ORIENTED_EDGE ( 'NONE', *, *, #9945, .T. ) ;
#11144=DIRECTION ( 'NONE',  ( -1.000000000000000000, -0.000000000000000000, -1.114413700119375779E-16 ) ) ;
#11147=ADVANCED_FACE ( 'NONE', ( #9704 ), #15859, .F. ) ;
#11149=ADVANCED_FACE ( 'NONE', ( #3886 ), #6404, .F. ) ;
#11153=CARTESIAN_POINT ( 'NONE',  ( 11.45098066423670247, 0.000000000000000000, 1.122567565269603304E-11 ) ) ;
#11157=ORIENTED_EDGE ( 'NONE', *, *, #1094, .F. ) ;
#11167=DIRECTION ( 'NONE',  ( 0.5000000000000002220, 0.000000000000000000, -0.8660254037844383745 ) ) ;
#11170=CARTESIAN_POINT ( 'NONE',  ( 4.790360200640285449, -4.342938577510797593, -48.50984154344460109 ) ) ;
#11171=ORIENTED_EDGE ( 'NONE', *, *, #6341, .F. ) ;
#11176=DIRECTION ( 'NONE',  ( -0.000000000000000000, -1.000000000000000000, -0.000000000000000000 ) ) ;
#11191=ORIENTED_EDGE ( 'NONE', *, *, #10910, .T. ) ;
#11211=DIRECTION ( 'NONE',  ( -0.000000000000000000, -1.000000000000000000, -0.000000000000000000 ) ) ;
#11231=DIRECTION ( 'NONE',  ( 0.8660254037844383745, 0.000000000000000000, 0.5000000000000004441 ) ) ;
#11241=EDGE_CURVE ( 'NONE', #10374, #12492, #1619, .T. ) ;
#11253=CARTESIAN_POINT ( 'NONE',  ( 3.007418566627519940, -3.000000000000001332, -48.95213768370648211 ) ) ;
#11255=CARTESIAN_POINT ( 'NONE',  ( 57.73502691896258199, -37.00000000000000711, 2.081668171172168513E-14 ) ) ;
#11259=EDGE_CURVE ( 'NONE', #395, #742, #13732, .T. ) ;
#11261=EDGE_CURVE ( 'NONE', #4540, #15603, #3619, .T. ) ;
#11268=CARTESIAN_POINT ( 'NONE',  ( -44.43375672972994295, -3.000000000000000000, -19.99999999999594635 ) ) ;
#11272=DIRECTION ( 'NONE',  ( 1.000000000000000000, 0.000000000000000000, 3.343241100358131282E-16 ) ) ;
#11281=VECTOR ( 'NONE', #9659, 1000.000000000000114 ) ;
#11283=ADVANCED_FACE ( 'NONE', ( #14234 ), #8103, .F. ) ;
#11285=AXIS2_PLACEMENT_3D ( 'NONE', #4959, #10063, #14993 ) ;
#11295=AXIS2_PLACEMENT_3D ( 'NONE', #13152, #11860, #2087 ) ;
#11298=ORIENTED_EDGE ( 'NONE', *, *, #4198, .F. ) ;
#11314=LINE ( 'NONE', #11625, #6013 ) ;
#11316=EDGE_CURVE ( 'NONE', #15369, #6220, #1785, .T. ) ;
#11317=VERTEX_POINT ( 'NONE', #4377 ) ;
#11321=VECTOR ( 'NONE', #8230, 1000.000000000000000 ) ;
#11334=LINE ( 'NONE', #6176, #233 ) ;
#11341=ORIENTED_EDGE ( 'NONE', *, *, #9020, .F. ) ;
#11350=FACE_OUTER_BOUND ( 'NONE', #1808, .T. ) ;
#11355=DIRECTION ( 'NONE',  ( -0.000000000000000000, 1.000000000000000000, 0.000000000000000000 ) ) ;
#11360=DIRECTION ( 'NONE',  ( -1.000000000000000000, 0.000000000000000000, 0.000000000000000000 ) ) ;
#11371=EDGE_CURVE ( 'NONE', #9071, #11683, #1954, .T. ) ;
#11378=FACE_OUTER_BOUND ( 'NONE', #7618, .T. ) ;
#11379=ORIENTED_EDGE ( 'NONE', *, *, #4253, .F. ) ;
#11393=ORIENTED_EDGE ( 'NONE', *, *, #7878, .F. ) ;
#11398=CARTESIAN_POINT ( 'NONE',  ( -28.86751345948126612, 0.000000000000000000, -18.00000000000000355 ) ) ;
#11410=CARTESIAN_POINT ( 'NONE',  ( -55.00000000000000000, 0.000000000000000000, 19.99999999999999289 ) ) ;
#11415=CIRCLE ( 'NONE', #13996, 2.649999999999985700 ) ;
#11417=AXIS2_PLACEMENT_3D ( 'NONE', #11752, #551, #14436 ) ;
#11430=DIRECTION ( 'NONE',  ( 0.000000000000000000, 0.000000000000000000, 1.000000000000000000 ) ) ;
#11437=EDGE_CURVE ( 'NONE', #7472, #482, #15638, .T. ) ;
#11453=CARTESIAN_POINT ( 'NONE',  ( -28.86751345948129455, 88.59290746114278647, 49.99999999999999289 ) ) ;
#11472=ORIENTED_EDGE ( 'NONE', *, *, #7153, .T. ) ;
#11473=CARTESIAN_POINT ( 'NONE',  ( -44.15702331412045822, -3.242827243955582084, 21.01093009162843117 ) ) ;
#11475=DIRECTION ( 'NONE',  ( 0.000000000000000000, 0.000000000000000000, -1.000000000000000000 ) ) ;
#11479=CARTESIAN_POINT ( 'NONE',  ( 57.73502691896258199, 0.000000000000000000, 2.081668171172168513E-14 ) ) ;
#11489=DIRECTION ( 'NONE',  ( -0.000000000000000000, -1.000000000000000000, -0.000000000000000000 ) ) ;
#11491=VECTOR ( 'NONE', #10116, 1000.000000000000114 ) ;
#11506=ADVANCED_FACE ( 'NONE', ( #3627 ), #7204, .F. ) ;
#11512=CARTESIAN_POINT ( 'NONE',  ( -21.01110699893060030, -3.000000000000001332, 33.74230484541325126 ) ) ;
#11520=DIRECTION ( 'NONE',  ( 0.000000000000000000, 0.000000000000000000, -1.000000000000000000 ) ) ;
#11527=ORIENTED_EDGE ( 'NONE', *, *, #13016, .T. ) ;
#11532=EDGE_CURVE ( 'NONE', #10685, #9400, #14778, .T. ) ;
#11555=EDGE_CURVE ( 'NONE', #14284, #13587, #923, .T. ) ;
#11557=EDGE_LOOP ( 'NONE', ( #5829, #12421, #2565, #13390 ) ) ;
#11560=CARTESIAN_POINT ( 'NONE',  ( 47.32050807568879947, -37.00000000000000711, -41.96152422706630603 ) ) ;
#11571=( NAMED_UNIT ( * ) PLANE_ANGLE_UNIT ( ) SI_UNIT ( $, .RADIAN. ) );
#11579=CIRCLE ( 'NONE', #4621, 28.00000000000000355 ) ;
#11584=LINE ( 'NONE', #7967, #7598 ) ;
#11601=CARTESIAN_POINT ( 'NONE',  ( 11.45098066423670247, -3.000000000000000000, 1.122567565269603304E-11 ) ) ;
#11619=EDGE_CURVE ( 'NONE', #2121, #7238, #10901, .T. ) ;
#11622=CARTESIAN_POINT ( 'NONE',  ( -44.32078660371288237, -3.761076017575719188, -20.42441216671174686 ) ) ;
#11625=CARTESIAN_POINT ( 'NONE',  ( -21.01110699893041911, -3.000000000000000000, -39.04230484541333368 ) ) ;
#11630=DIRECTION ( 'NONE',  ( -0.000000000000000000, 1.000000000000000000, -0.000000000000000000 ) ) ;
#11645=CARTESIAN_POINT ( 'NONE',  ( -21.01110699893060030, -3.000000000000000000, 36.39230484541324273 ) ) ;
#11666=ORIENTED_EDGE ( 'NONE', *, *, #12683, .T. ) ;
#11677=DIRECTION ( 'NONE',  ( -0.5000000000000004441, 0.000000000000000000, 0.8660254037844383745 ) ) ;
#11682=ORIENTED_EDGE ( 'NONE', *, *, #9945, .F. ) ;
#11683=VERTEX_POINT ( 'NONE', #4020 ) ;
#11685=ORIENTED_EDGE ( 'NONE', *, *, #13427, .T. ) ;
#11688=CARTESIAN_POINT ( 'NONE',  ( 14.41154273188013590, 88.59290746114278647, -60.96152422706631313 ) ) ;
#11703=VERTEX_POINT ( 'NONE', #7518 ) ;
#11709=VERTEX_POINT ( 'NONE', #15189 ) ;
#11743=ORIENTED_EDGE ( 'NONE', *, *, #10910, .F. ) ;
#11745=EDGE_LOOP ( 'NONE', ( #9654, #6902, #2722, #15567 ) ) ;
#11752=CARTESIAN_POINT ( 'NONE',  ( -5.725490332117410652, -3.000000000000000000, 9.916840153471811803 ) ) ;
#11760=VECTOR ( 'NONE', #14514, 1000.000000000000000 ) ;
#11762=DIRECTION ( 'NONE',  ( 0.000000000000000000, 0.000000000000000000, -1.000000000000000000 ) ) ;
#11764=ORIENTED_EDGE ( 'NONE', *, *, #4257, .F. ) ;
#11773=CARTESIAN_POINT ( 'NONE',  ( 2.875844205642646756, -3.000000000000000000, 48.98110827882563711 ) ) ;
#11783=LINE ( 'NONE', #6637, #12515 ) ;
#11802=ORIENTED_EDGE ( 'NONE', *, *, #925, .F. ) ;
#11807=CIRCLE ( 'NONE', #5380, 39.99999999999999289 ) ;
#11812=EDGE_CURVE ( 'NONE', #13331, #7289, #14863, .T. ) ;
#11814=ADVANCED_FACE ( 'NONE', ( #11378 ), #6383, .T. ) ;
#11819=ORIENTED_EDGE ( 'NONE', *, *, #6445, .F. ) ;
#11822=CIRCLE ( 'NONE', #4871, 40.00000000000001421 ) ;
#11830=VECTOR ( 'NONE', #2953, 1000.000000000000114 ) ;
#11837=DIRECTION ( 'NONE',  ( 0.000000000000000000, -1.000000000000000000, 0.000000000000000000 ) ) ;
#11844=VECTOR ( 'NONE', #9476, 1000.000000000000114 ) ;
#11853=EDGE_CURVE ( 'NONE', #5239, #1848, #8005, .T. ) ;
#11855=CARTESIAN_POINT ( 'NONE',  ( 3.876648187198773687, -3.253774389711713511, 48.74739051362634257 ) ) ;
#11860=DIRECTION ( 'NONE',  ( 0.000000000000000000, 1.000000000000000000, 0.000000000000000000 ) ) ;
#11884=VERTEX_POINT ( 'NONE', #797 ) ;
#11897=CARTESIAN_POINT ( 'NONE',  ( 0.000000000000000000, 0.000000000000000000, 0.000000000000000000 ) ) ;
#11898=ORIENTED_EDGE ( 'NONE', *, *, #9462, .F. ) ;
#11932=CARTESIAN_POINT ( 'NONE',  ( 33.48631561300354065, -3.000000000000000000, 14.00000000000909850 ) ) ;
#11949=DIRECTION ( 'NONE',  ( -0.000000000000000000, 1.000000000000000000, -0.000000000000000000 ) ) ;
#11955=CARTESIAN_POINT ( 'NONE',  ( -21.01110699893060030, 0.000000000000000000, 39.04230484541323420 ) ) ;
#11956=EDGE_LOOP ( 'NONE', ( #12693, #5556, #6880, #12814 ) ) ;
#11959=LINE ( 'NONE', #10451, #4886 ) ;
#11969=DIRECTION ( 'NONE',  ( -0.5000000000000000000, 8.673617379884033500E-16, 0.8660254037844385966 ) ) ;
#11970=ORIENTED_EDGE ( 'NONE', *, *, #4198, .T. ) ;
#11972=DIRECTION ( 'NONE',  ( 0.000000000000000000, 0.000000000000000000, 1.000000000000000000 ) ) ;
#11977=ORIENTED_EDGE ( 'NONE', *, *, #6445, .T. ) ;
#11979=CARTESIAN_POINT ( 'NONE',  ( -60.00000000000000000, -5.000000000000000000, -20.00000000000000711 ) ) ;
#11985=CARTESIAN_POINT ( 'NONE',  ( 33.48631561299831105, -3.000000000000000000, -13.99999999999999645 ) ) ;
#11987=DIRECTION ( 'NONE',  ( 0.000000000000000000, -1.000000000000000000, 0.000000000000000000 ) ) ;
#12010=PLANE ( 'NONE',  #6566 ) ;
#12038=ORIENTED_EDGE ( 'NONE', *, *, #15692, .T. ) ;
#12039=PRODUCT_DEFINITION_FORMATION_WITH_SPECIFIED_SOURCE ( 'ANY', '', #10551, .NOT_KNOWN. ) ;
#12047=ADVANCED_FACE ( 'NONE', ( #15668 ), #7416, .T. ) ;
#12052=VECTOR ( 'NONE', #12987, 1000.000000000000114 ) ;
#12064=B_SPLINE_CURVE_WITH_KNOTS ( 'NONE', 3,
 ( #10621, #682, #5607, #10547, #9328, #7228, #3570, #14890, #9951, #2193, #6246, #1301, #7463, #4943, #12284, #103 ),
 .UNSPECIFIED., .F., .F.,
 ( 4, 2, 2, 2, 2, 2, 2, 4 ),
 ( 6.534274128967059438E-16, 0.0003988053453845139722, 0.0007976106907683744958, 0.001196416036152234911, 0.001595221381536094350, 0.002392832072303797616, 0.002791637417687638408, 0.003190442763071479632 ),
 .UNSPECIFIED. ) ;
#12080=CIRCLE ( 'NONE', #5149, 2.649999999999992806 ) ;
#12088=FACE_OUTER_BOUND ( 'NONE', #4782, .T. ) ;
#12089=VECTOR ( 'NONE', #9782, 1000.000000000000114 ) ;
#12102=ORIENTED_EDGE ( 'NONE', *, *, #9664, .T. ) ;
#12105=DIRECTION ( 'NONE',  ( 0.000000000000000000, -1.000000000000000000, 0.000000000000000000 ) ) ;
#12107=CYLINDRICAL_SURFACE ( 'NONE', #162, 2.649999999999992806 ) ;
#12108=VECTOR ( 'NONE', #9963, 1000.000000000000000 ) ;
#12112=CARTESIAN_POINT ( 'NONE',  ( -44.43375672972994295, -5.000000000000000000, -20.00000000000000355 ) ) ;
#12138=EDGE_LOOP ( 'NONE', ( #4501, #2704, #7277, #7940, #15076, #75, #5539, #2050, #1327, #11666, #8409, #12292 ) ) ;
#12141=EDGE_CURVE ( 'NONE', #13521, #2457, #3441, .T. ) ;
#12157=ORIENTED_EDGE ( 'NONE', *, *, #2547, .T. ) ;
#12161=DIRECTION ( 'NONE',  ( -0.000000000000000000, 1.000000000000000000, -0.000000000000000000 ) ) ;
#12164=DIRECTION ( 'NONE',  ( -0.000000000000000000, 1.000000000000000000, -0.000000000000000000 ) ) ;
#12170=ORIENTED_EDGE ( 'NONE', *, *, #905, .T. ) ;
#12180=AXIS2_PLACEMENT_3D ( 'NONE', #14274, #10641, #1745 ) ;
#12189=AXIS2_PLACEMENT_3D ( 'NONE', #5983, #8653, #8578 ) ;
#12191=EDGE_CURVE ( 'NONE', #4347, #11118, #947, .T. ) ;
#12206=ADVANCED_FACE ( 'NONE', ( #9903 ), #13862, .F. ) ;
#12214=ORIENTED_EDGE ( 'NONE', *, *, #10856, .T. ) ;
#12216=DIRECTION ( 'NONE',  ( 0.000000000000000000, -0.000000000000000000, -1.000000000000000000 ) ) ;
#12218=DIRECTION ( 'NONE',  ( -0.000000000000000000, 1.000000000000000000, -0.000000000000000000 ) ) ;
#12229=CARTESIAN_POINT ( 'NONE',  ( 33.48631561299828974, -4.999999999999997335, 14.00000000000001243 ) ) ;
#12232=EDGE_LOOP ( 'NONE', ( #11191, #14946, #6727, #3739, #14683, #10955, #1370 ) ) ;
#12262=DIRECTION ( 'NONE',  ( 0.000000000000000000, 0.000000000000000000, 1.000000000000000000 ) ) ;
#12265=AXIS2_PLACEMENT_3D ( 'NONE', #4996, #11069, #6056 ) ;
#12284=CARTESIAN_POINT ( 'NONE',  ( 40.89008552033507726, -3.000000000000000444, 27.08056972037525867 ) ) ;
#12292=ORIENTED_EDGE ( 'NONE', *, *, #8722, .T. ) ;
#12293=CARTESIAN_POINT ( 'NONE',  ( -28.86751345948130165, -35.00000000000000000, 17.99999999999999645 ) ) ;
#12316=VERTEX_POINT ( 'NONE', #2628 ) ;
#12318=ORIENTED_EDGE ( 'NONE', *, *, #11853, .F. ) ;
#12335=ORIENTED_EDGE ( 'NONE', *, *, #1176, .F. ) ;
#12353=CARTESIAN_POINT ( 'NONE',  ( -1.154700538379222596, 0.000000000000000000, -34.00000000000000000 ) ) ;
#12358=LINE ( 'NONE', #4774, #9132 ) ;
#12368=FACE_OUTER_BOUND ( 'NONE', #9308, .T. ) ;
#12374=CARTESIAN_POINT ( 'NONE',  ( 3.520694248372895352, -3.098194602941630738, -48.83371901636445500 ) ) ;
#12378=DIRECTION ( 'NONE',  ( 0.5000000000000005551, 0.000000000000000000, -0.8660254037844382635 ) ) ;
#12380=ORIENTED_EDGE ( 'NONE', *, *, #5627, .T. ) ;
#12384=CARTESIAN_POINT ( 'NONE',  ( 4.896370289181586344, -3.000000000000000000, 48.48076211353308906 ) ) ;
#12396=ORIENTED_EDGE ( 'NONE', *, *, #3559, .F. ) ;
#12403=CARTESIAN_POINT ( 'NONE',  ( -44.43375672974056556, -5.000000000000000000, 19.99999999999999645 ) ) ;
#12421=ORIENTED_EDGE ( 'NONE', *, *, #15462, .T. ) ;
#12422=DIRECTION ( 'NONE',  ( 0.000000000000000000, 0.000000000000000000, 1.000000000000000000 ) ) ;
#12423=VECTOR ( 'NONE', #10994, 1000.000000000000114 ) ;
#12434=DIRECTION ( 'NONE',  ( 0.000000000000000000, 0.000000000000000000, 1.000000000000000000 ) ) ;
#12444=VECTOR ( 'NONE', #13087, 1000.000000000000000 ) ;
#12454=EDGE_LOOP ( 'NONE', ( #8989, #5836, #7953, #7433 ) ) ;
#12460=AXIS2_PLACEMENT_3D ( 'NONE', #5552, #7011, #8149 ) ;
#12467=AXIS2_PLACEMENT_3D ( 'NONE', #1724, #536, #2047 ) ;
#12468=ORIENTED_EDGE ( 'NONE', *, *, #10861, .F. ) ;
#12469=LINE ( 'NONE', #1408, #9738 ) ;
#12473=ORIENTED_EDGE ( 'NONE', *, *, #13958, .F. ) ;
#12492=VERTEX_POINT ( 'NONE', #7461 ) ;
#12495=DIRECTION ( 'NONE',  ( -0.000000000000000000, 0.000000000000000000, 1.000000000000000000 ) ) ;
#12496=ORIENTED_EDGE ( 'NONE', *, *, #8002, .T. ) ;
#12498=PLANE ( 'NONE',  #7732 ) ;
#12512=ORIENTED_EDGE ( 'NONE', *, *, #12683, .F. ) ;
#12515=VECTOR ( 'NONE', #12834, 1000.000000000000000 ) ;
#12518=AXIS2_PLACEMENT_3D ( 'NONE', #14642, #3565, #8992 ) ;
#12528=CARTESIAN_POINT ( 'NONE',  ( -60.00000000000000000, -35.00000000000000000, -18.00000000000000000 ) ) ;
#12532=ORIENTED_EDGE ( 'NONE', *, *, #1622, .F. ) ;
#12533=CYLINDRICAL_SURFACE ( 'NONE', #10794, 2.649999999999992806 ) ;
#12538=VECTOR ( 'NONE', #14260, 1000.000000000000000 ) ;
#12543=DIRECTION ( 'NONE',  ( 0.5000000000000001110, 0.000000000000000000, -0.8660254037844384856 ) ) ;
#12562=CARTESIAN_POINT ( 'NONE',  ( 2.875844205642646756, -3.000000000000000000, 48.98110827882563711 ) ) ;
#12582=EDGE_LOOP ( 'NONE', ( #15488, #12214, #9131, #5058 ) ) ;
#12588=DIRECTION ( 'NONE',  ( 0.000000000000000000, 0.000000000000000000, -1.000000000000000000 ) ) ;
#12598=EDGE_CURVE ( 'NONE', #2379, #10415, #5773, .T. ) ;
#12599=ORIENTED_EDGE ( 'NONE', *, *, #15815, .T. ) ;
#12607=DIRECTION ( 'NONE',  ( 0.000000000000000000, 1.000000000000000000, 0.000000000000000000 ) ) ;
#12621=VERTEX_POINT ( 'NONE', #7296 ) ;
#12667=CARTESIAN_POINT ( 'NONE',  ( -44.01347164682042035, -3.060691311048526764, -21.49473191792460014 ) ) ;
#12675=ORIENTED_EDGE ( 'NONE', *, *, #10856, .F. ) ;
#12679=LINE ( 'NONE', #11560, #5086 ) ;
#12680=DIRECTION ( 'NONE',  ( 0.000000000000000000, 0.000000000000000000, -1.000000000000000000 ) ) ;
#12683=EDGE_CURVE ( 'NONE', #7238, #10747, #12679, .T. ) ;
#12688=EDGE_LOOP ( 'NONE', ( #9166, #1647, #14258, #12955 ) ) ;
#12691=LINE ( 'NONE', #1634, #14692 ) ;
#12693=ORIENTED_EDGE ( 'NONE', *, *, #7074, .T. ) ;
#12697=CIRCLE ( 'NONE', #6783, 4.999999999999997335 ) ;
#12708=CARTESIAN_POINT ( 'NONE',  ( -21.01110699893041911, 0.000000000000000000, -36.39230484541334221 ) ) ;
#12720=ADVANCED_FACE ( 'NONE', ( #7619 ), #8994, .T. ) ;
#12732=ORIENTED_EDGE ( 'NONE', *, *, #2709, .T. ) ;
#12752=VERTEX_POINT ( 'NONE', #8831 ) ;
#12753=VERTEX_POINT ( 'NONE', #11398 ) ;
#12756=CARTESIAN_POINT ( 'NONE',  ( -44.43375672974056556, -5.000000000000000000, 19.99999999999999645 ) ) ;
#12767=ORIENTED_EDGE ( 'NONE', *, *, #4185, .F. ) ;
#12768=SURFACE_STYLE_FILL_AREA ( #9008 ) ;
#12773=ORIENTED_EDGE ( 'NONE', *, *, #4639, .T. ) ;
#12792=VECTOR ( 'NONE', #6441, 1000.000000000000000 ) ;
#12807=DIRECTION ( 'NONE',  ( 0.000000000000000000, 0.000000000000000000, -1.000000000000000000 ) ) ;
#12809=AXIS2_PLACEMENT_3D ( 'NONE', #13569, #13415, #13251 ) ;
#12814=ORIENTED_EDGE ( 'NONE', *, *, #2079, .T. ) ;
#12821=ORIENTED_EDGE ( 'NONE', *, *, #7708, .T. ) ;
#12834=DIRECTION ( 'NONE',  ( 0.000000000000000000, -1.000000000000000000, 0.000000000000000000 ) ) ;
#12842=EDGE_CURVE ( 'NONE', #12621, #1848, #9542, .T. ) ;
#12857=CIRCLE ( 'NONE', #3566, 5.000000000000000888 ) ;
#12866=VECTOR ( 'NONE', #12981, 1000.000000000000000 ) ;
#12880=VERTEX_POINT ( 'NONE', #5668 ) ;
#12886=DIRECTION ( 'NONE',  ( 0.000000000000000000, 0.000000000000000000, 1.000000000000000000 ) ) ;
#12887=CYLINDRICAL_SURFACE ( 'NONE', #12180, 2.000000000000001776 ) ;
#12888=CYLINDRICAL_SURFACE ( 'NONE', #14432, 32.00000000000000711 ) ;
#12897=ORIENTED_EDGE ( 'NONE', *, *, #2316, .T. ) ;
#12904=CARTESIAN_POINT ( 'NONE',  ( 57.73502691896258199, 88.59290746114278647, 2.081668171172168513E-14 ) ) ;
#12910=CYLINDRICAL_SURFACE ( 'NONE', #6283, 2.649999999999992806 ) ;
#12923=DIRECTION ( 'NONE',  ( 1.114413700119375779E-16, -0.000000000000000000, -1.000000000000000000 ) ) ;
#12924=CARTESIAN_POINT ( 'NONE',  ( 40.04621312669365807, -3.477892933143086562, -27.97002203198492865 ) ) ;
#12927=EDGE_CURVE ( 'NONE', #4347, #10581, #15690, .T. ) ;
#12929=EDGE_CURVE ( 'NONE', #15266, #13331, #2983, .T. ) ;
#12931=ADVANCED_FACE ( 'NONE', ( #1857 ), #5588, .T. ) ;
#12955=ORIENTED_EDGE ( 'NONE', *, *, #11241, .F. ) ;
#12962=CARTESIAN_POINT ( 'NONE',  ( 14.41154273188013590, -35.00000000000000000, -60.96152422706631313 ) ) ;
#12974=VERTEX_POINT ( 'NONE', #2480 ) ;
#12981=DIRECTION ( 'NONE',  ( -1.000000000000000000, -0.000000000000000000, -3.343241100358131282E-16 ) ) ;
#12983=CARTESIAN_POINT ( 'NONE',  ( 57.73502691896258199, -37.00000000000000711, 2.081668171172168513E-14 ) ) ;
#12987=DIRECTION ( 'NONE',  ( -0.4999999999999998335, -0.000000000000000000, -0.8660254037844387076 ) ) ;
#12993=VERTEX_POINT ( 'NONE', #7278 ) ;
#12997=DIRECTION ( 'NONE',  ( 0.8660254037844381525, 0.000000000000000000, 0.5000000000000007772 ) ) ;
#12999=DIRECTION ( 'NONE',  ( 1.000000000000000000, 0.000000000000000000, 0.000000000000000000 ) ) ;
#13010=ORIENTED_EDGE ( 'NONE', *, *, #534, .F. ) ;
#13015=ADVANCED_FACE ( 'NONE', ( #2253 ), #13463, .F. ) ;
#13016=EDGE_CURVE ( 'NONE', #7869, #15369, #8174, .T. ) ;
#13021=STYLED_ITEM ( 'NONE', ( #13833 ), #1740 ) ;
#13025=DIRECTION ( 'NONE',  ( 0.000000000000000000, -1.000000000000000000, 0.000000000000000000 ) ) ;
#13027=ORIENTED_EDGE ( 'NONE', *, *, #11532, .T. ) ;
#13040=AXIS2_PLACEMENT_3D ( 'NONE', #1297, #13330, #6243 ) ;
#13052=UNCERTAINTY_MEASURE_WITH_UNIT (LENGTH_MEASURE( 1.000000000000000082E-05 ), #5255, 'distance_accuracy_value', 'NONE');
#13066=CARTESIAN_POINT ( 'NONE',  ( 3.136976819694406782, -3.012271619929380417, 48.92291361451623999 ) ) ;
#13076=ADVANCED_FACE ( 'NONE', ( #8734 ), #12107, .F. ) ;
#13083=DIRECTION ( 'NONE',  ( 0.000000000000000000, 1.000000000000000000, 0.000000000000000000 ) ) ;
#13087=DIRECTION ( 'NONE',  ( -0.000000000000000000, 1.000000000000000000, -0.000000000000000000 ) ) ;
#13093=CIRCLE ( 'NONE', #2252, 2.649999999999992806 ) ;
#13120=CARTESIAN_POINT ( 'NONE',  ( -28.86751345948126612, -3.000000000000000000, -22.00000000000000711 ) ) ;
#13126=DIRECTION ( 'NONE',  ( 0.000000000000000000, 0.000000000000000000, 1.000000000000000000 ) ) ;
#13127=CARTESIAN_POINT ( 'NONE',  ( 47.32050807568879947, -4.999999999999997335, -41.96152422706630603 ) ) ;
#13131=DIRECTION ( 'NONE',  ( -0.000000000000000000, 1.000000000000000000, -0.000000000000000000 ) ) ;
#13140=ORIENTED_EDGE ( 'NONE', *, *, #2709, .F. ) ;
#13152=CARTESIAN_POINT ( 'NONE',  ( -21.01110699893041911, 0.000000000000000000, -36.39230484541334221 ) ) ;
#13201=CARTESIAN_POINT ( 'NONE',  ( -1.154700538379222596, 88.59290746114278647, -34.00000000000000000 ) ) ;
#13211=DIRECTION ( 'NONE',  ( 0.000000000000000000, 0.000000000000000000, -1.000000000000000000 ) ) ;
#13216=CARTESIAN_POINT ( 'NONE',  ( 12.67949192431126093, -37.00000000000000711, -61.96152422706632024 ) ) ;
#13220=CARTESIAN_POINT ( 'NONE',  ( 0.000000000000000000, 0.000000000000000000, 0.000000000000000000 ) ) ;
#13235=EDGE_CURVE ( 'NONE', #4642, #7472, #10503, .T. ) ;
#13242=DIRECTION ( 'NONE',  ( -1.114413700119375779E-16, -0.000000000000000000, 1.000000000000000000 ) ) ;
#13244=PLANE ( 'NONE',  #13335 ) ;
#13251=DIRECTION ( 'NONE',  ( 0.000000000000000000, 0.000000000000000000, 1.000000000000000000 ) ) ;
#13256=DIRECTION ( 'NONE',  ( 0.000000000000000000, 0.000000000000000000, 1.000000000000000000 ) ) ;
#13268=TOROIDAL_SURFACE ( 'NONE', #14067, 28.00000000000000355, 2.000000000000000000 ) ;
#13291=CARTESIAN_POINT ( 'NONE',  ( 30.02221399786052913, 0.000000000000000000, 16.00000000000001066 ) ) ;
#13293=AXIS2_PLACEMENT_3D ( 'NONE', #12229, #1168, #11040 ) ;
#13296=CARTESIAN_POINT ( 'NONE',  ( 47.32050807568875683, -35.00000000000000000, 41.96152422706633445 ) ) ;
#13300=ORIENTED_EDGE ( 'NONE', *, *, #13516, .F. ) ;
#13302=ORIENTED_EDGE ( 'NONE', *, *, #9664, .F. ) ;
#13304=ADVANCED_FACE ( 'NONE', ( #9441 ), #8083, .T. ) ;
#13305=DIRECTION ( 'NONE',  ( 0.000000000000000000, 1.000000000000000000, 0.000000000000000000 ) ) ;
#13318=CIRCLE ( 'NONE', #1465, 29.99999999999999289 ) ;
#13330=DIRECTION ( 'NONE',  ( 0.000000000000000000, -1.000000000000000000, 0.000000000000000000 ) ) ;
#13331=VERTEX_POINT ( 'NONE', #15351 ) ;
#13335=AXIS2_PLACEMENT_3D ( 'NONE', #8193, #6978, #2344 ) ;
#13341=CARTESIAN_POINT ( 'NONE',  ( -28.86751345948126257, 0.000000000000000000, -50.00000000000000711 ) ) ;
#13351=VECTOR ( 'NONE', #3415, 1000.000000000000000 ) ;
#13357=DIRECTION ( 'NONE',  ( 0.8660254037844387076, 0.000000000000000000, -0.4999999999999998335 ) ) ;
#13361=VECTOR ( 'NONE', #12543, 1000.000000000000227 ) ;
#13380=EDGE_CURVE ( 'NONE', #7223, #715, #14846, .T. ) ;
#13390=ORIENTED_EDGE ( 'NONE', *, *, #12927, .F. ) ;
#13393=CARTESIAN_POINT ( 'NONE',  ( 12.67949192431126093, -37.00000000000000711, -61.96152422706632024 ) ) ;
#13402=FACE_BOUND ( 'NONE', #8802, .T. ) ;
#13415=DIRECTION ( 'NONE',  ( 0.000000000000000000, 1.000000000000000000, 0.000000000000000000 ) ) ;
#13427=EDGE_CURVE ( 'NONE', #15871, #4627, #5021, .T. ) ;
#13439=ORIENTED_EDGE ( 'NONE', *, *, #10875, .F. ) ;
#13460=DIRECTION ( 'NONE',  ( -1.000000000000000000, 0.000000000000000000, -3.343241100358131282E-16 ) ) ;
#13463=PLANE ( 'NONE',  #8428 ) ;
#13470=LINE ( 'NONE', #4856, #12089 ) ;
#13473=AXIS2_PLACEMENT_3D ( 'NONE', #15492, #4646, #3193 ) ;
#13515=PLANE ( 'NONE',  #14348 ) ;
#13516=EDGE_CURVE ( 'NONE', #9104, #482, #10455, .T. ) ;
#13521=VERTEX_POINT ( 'NONE', #15009 ) ;
#13532=DIRECTION ( 'NONE',  ( 0.4999999999999998335, 0.000000000000000000, 0.8660254037844387076 ) ) ;
#13566=ORIENTED_EDGE ( 'NONE', *, *, #4725, .T. ) ;
#13569=CARTESIAN_POINT ( 'NONE',  ( -21.01110699893060030, 0.000000000000000000, 36.39230484541324273 ) ) ;
#13570=ADVANCED_FACE ( 'NONE', ( #7823 ), #6601, .F. ) ;
#13581=CARTESIAN_POINT ( 'NONE',  ( 4.896370289182463864, -4.865128266864630291, -48.48076211353469489 ) ) ;
#13587=VERTEX_POINT ( 'NONE', #6284 ) ;
#13590=CARTESIAN_POINT ( 'NONE',  ( -21.01110699893041911, -3.000000000000000000, -36.39230484541334221 ) ) ;
#13599=DIRECTION ( 'NONE',  ( 0.000000000000000000, 0.000000000000000000, -1.000000000000000000 ) ) ;
#13609=VERTEX_POINT ( 'NONE', #12562 ) ;
#13620=EDGE_CURVE ( 'NONE', #8118, #10581, #3725, .T. ) ;
#13621=CARTESIAN_POINT ( 'NONE',  ( -28.86751345948126612, -4.999999999999997335, -20.00000000000000355 ) ) ;
#13633=FACE_OUTER_BOUND ( 'NONE', #8114, .T. ) ;
#13637=VERTEX_POINT ( 'NONE', #6365 ) ;
#13649=CARTESIAN_POINT ( 'NONE',  ( -60.00000000000000000, -35.00000000000000000, 19.99999999999999289 ) ) ;
#13655=ORIENTED_EDGE ( 'NONE', *, *, #5000, .T. ) ;
#13658=ORIENTED_EDGE ( 'NONE', *, *, #11261, .T. ) ;
#13659=CARTESIAN_POINT ( 'NONE',  ( 39.53738644056436868, -5.000000000000000000, 28.48076211354233322 ) ) ;
#13664=DIRECTION ( 'NONE',  ( 0.8660254037844388186, -0.000000000000000000, -0.4999999999999998890 ) ) ;
#13709=ORIENTED_EDGE ( 'NONE', *, *, #1176, .T. ) ;
#13724=DIRECTION ( 'NONE',  ( -0.000000000000000000, -1.000000000000000000, -0.000000000000000000 ) ) ;
#13731=AXIS2_PLACEMENT_3D ( 'NONE', #12983, #6867, #4509 ) ;
#13732=LINE ( 'NONE', #5186, #11491 ) ;
#13733=EDGE_CURVE ( 'NONE', #12492, #1994, #7876, .T. ) ;
#13741=CYLINDRICAL_SURFACE ( 'NONE', #8488, 5.000000000000001776 ) ;
#13756=AXIS2_PLACEMENT_3D ( 'NONE', #6932, #11677, #9199 ) ;
#13758=CARTESIAN_POINT ( 'NONE',  ( 47.32050807568879947, 0.000000000000000000, -41.96152422706630603 ) ) ;
#13773=CARTESIAN_POINT ( 'NONE',  ( 42.02221399786069611, -3.000000000000001332, 1.040834085586084257E-13 ) ) ;
#13787=EDGE_LOOP ( 'NONE', ( #1615, #12335, #6746, #13655, #11977 ) ) ;
#13794=CARTESIAN_POINT ( 'NONE',  ( 11.45098066423670247, -3.000000000000000000, 1.122567565269603304E-11 ) ) ;
#13800=CARTESIAN_POINT ( 'NONE',  ( -44.05083158856042047, -3.097286126993890942, -21.37039199565628067 ) ) ;
#13812=CARTESIAN_POINT ( 'NONE',  ( -44.41643093307008172, -4.472255266399358220, 20.06631602343790632 ) ) ;
#13815=DIRECTION ( 'NONE',  ( -0.5000000000000005551, 0.000000000000000000, 0.8660254037844382635 ) ) ;
#13817=VECTOR ( 'NONE', #6864, 1000.000000000000000 ) ;
#13833=PRESENTATION_STYLE_ASSIGNMENT (( #4137 ) ) ;
#13836=DIRECTION ( 'NONE',  ( -0.000000000000000000, 1.000000000000000000, -0.000000000000000000 ) ) ;
#13852=DIRECTION ( 'NONE',  ( 1.000000000000000000, 0.000000000000000000, 0.000000000000000000 ) ) ;
#13861=FACE_OUTER_BOUND ( 'NONE', #4304, .T. ) ;
#13862=PLANE ( 'NONE',  #699 ) ;
#13864=AXIS2_PLACEMENT_3D ( 'NONE', #9279, #9350, #9428 ) ;
#13893=CIRCLE ( 'NONE', #14121, 2.649999999999985700 ) ;
#13908=EDGE_CURVE ( 'NONE', #11317, #15266, #15737, .T. ) ;
#13922=EDGE_CURVE ( 'NONE', #621, #5426, #14663, .T. ) ;
#13951=ORIENTED_EDGE ( 'NONE', *, *, #14643, .F. ) ;
#13957=DIRECTION ( 'NONE',  ( 0.000000000000000000, -1.000000000000000000, 0.000000000000000000 ) ) ;
#13958=EDGE_CURVE ( 'NONE', #10113, #4642, #2297, .T. ) ;
#13978=VECTOR ( 'NONE', #3502, 1000.000000000000114 ) ;
#13979=ORIENTED_EDGE ( 'NONE', *, *, #991, .T. ) ;
#13990=EDGE_CURVE ( 'NONE', #6220, #560, #3742, .T. ) ;
#13991=SURFACE_SIDE_STYLE ('',( #12768 ) ) ;
#13995=ORIENTED_EDGE ( 'NONE', *, *, #534, .T. ) ;
#13996=AXIS2_PLACEMENT_3D ( 'NONE', #15126, #4045, #12680 ) ;
#14022=CARTESIAN_POINT ( 'NONE',  ( -28.86751345948126612, -37.00000000000000711, -20.00000000000000355 ) ) ;
#14028=DIRECTION ( 'NONE',  ( 1.000000000000000000, -0.000000000000000000, 1.114413700119375779E-16 ) ) ;
#14031=ADVANCED_FACE ( 'NONE', ( #1638 ), #1317, .F. ) ;
#14048=FACE_OUTER_BOUND ( 'NONE', #7676, .T. ) ;
#14064=DIRECTION ( 'NONE',  ( -1.114413700119375779E-16, 0.000000000000000000, 1.000000000000000000 ) ) ;
#14067=AXIS2_PLACEMENT_3D ( 'NONE', #7816, #5459, #11430 ) ;
#14079=STYLED_ITEM ( 'NONE', ( #178 ), #14760 ) ;
#14080=EDGE_LOOP ( 'NONE', ( #12732, #10009, #7855, #8708, #10169, #14659, #12473 ) ) ;
#14081=FACE_OUTER_BOUND ( 'NONE', #14251, .T. ) ;
#14114=AXIS2_PLACEMENT_3D ( 'NONE', #14602, #9524, #8324 ) ;
#14115=FACE_OUTER_BOUND ( 'NONE', #10669, .T. ) ;
#14117=FACE_OUTER_BOUND ( 'NONE', #891, .T. ) ;
#14118=LINE ( 'NONE', #7991, #8229 ) ;
#14119=DIRECTION ( 'NONE',  ( 0.8660254037844384856, -0.000000000000000000, 0.5000000000000004441 ) ) ;
#14121=AXIS2_PLACEMENT_3D ( 'NONE', #15811, #3748, #13599 ) ;
#14124=EDGE_LOOP ( 'NONE', ( #14409, #4238, #4677, #5567 ) ) ;
#14131=AXIS2_PLACEMENT_3D ( 'NONE', #1748, #7905, #6695 ) ;
#14141=CARTESIAN_POINT ( 'NONE',  ( -44.24585618745123128, -3.477892933143074572, -20.69602687709009459 ) ) ;
#14146=ORIENTED_EDGE ( 'NONE', *, *, #11371, .T. ) ;
#14154=DIRECTION ( 'NONE',  ( 0.000000000000000000, 0.000000000000000000, 1.000000000000000000 ) ) ;
#14164=VECTOR ( 'NONE', #3730, 1000.000000000000114 ) ;
#14173=ORIENTED_EDGE ( 'NONE', *, *, #1622, .T. ) ;
#14176=ORIENTED_EDGE ( 'NONE', *, *, #475, .T. ) ;
#14187=DIRECTION ( 'NONE',  ( 1.000000000000000000, 0.000000000000000000, 3.343241100358131282E-16 ) ) ;
#14191=ORIENTED_EDGE ( 'NONE', *, *, #11555, .T. ) ;
#14192=DIRECTION ( 'NONE',  ( -0.4999999999999997224, 0.000000000000000000, -0.8660254037844388186 ) ) ;
#14226=ORIENTED_EDGE ( 'NONE', *, *, #3559, .T. ) ;
#14233=CARTESIAN_POINT ( 'NONE',  ( 57.73502691896258199, -3.000000000000000000, 2.081668171172168513E-14 ) ) ;
#14234=FACE_OUTER_BOUND ( 'NONE', #2600, .T. ) ;
#14251=EDGE_LOOP ( 'NONE', ( #12675, #3751, #14837, #2665 ) ) ;
#14258=ORIENTED_EDGE ( 'NONE', *, *, #13733, .F. ) ;
#14259=FACE_OUTER_BOUND ( 'NONE', #15583, .T. ) ;
#14260=DIRECTION ( 'NONE',  ( -0.000000000000000000, 0.000000000000000000, 1.000000000000000000 ) ) ;
#14267=EDGE_LOOP ( 'NONE', ( #11099, #8941, #1781, #3029 ) ) ;
#14274=CARTESIAN_POINT ( 'NONE',  ( -5.725490332106779157, -5.000000000000000000, -22.00000000000000000 ) ) ;
#14283=LINE ( 'NONE', #3206, #9204 ) ;
#14284=VERTEX_POINT ( 'NONE', #10691 ) ;
#14309=CARTESIAN_POINT ( 'NONE',  ( -5.725490332117410652, -3.000000000000000000, 9.916840153471811803 ) ) ;
#14310=CARTESIAN_POINT ( 'NONE',  ( -44.43375672974056556, -3.000000000000000000, 19.99999999999999645 ) ) ;
#14317=VECTOR ( 'NONE', #12216, 1000.000000000000000 ) ;
#14339=DIRECTION ( 'NONE',  ( 0.000000000000000000, 0.000000000000000000, -1.000000000000000000 ) ) ;
#14348=AXIS2_PLACEMENT_3D ( 'NONE', #2453, #4816, #8549 ) ;
#14373=CARTESIAN_POINT ( 'NONE',  ( 4.199643060765958502, -3.477892933143082121, 48.66604890908090653 ) ) ;
#14379=FACE_BOUND ( 'NONE', #15102, .T. ) ;
#14397=CARTESIAN_POINT ( 'NONE',  ( 39.84845309559526072, -3.761076017575720964, -28.17072103117275716 ) ) ;
#14409=ORIENTED_EDGE ( 'NONE', *, *, #183, .T. ) ;
#14424=ADVANCED_FACE ( 'NONE', ( #9549 ), #14477, .F. ) ;
#14429=VERTEX_POINT ( 'NONE', #4096 ) ;
#14432=AXIS2_PLACEMENT_3D ( 'NONE', #784, #11837, #11520 ) ;
#14436=DIRECTION ( 'NONE',  ( 0.000000000000000000, 0.000000000000000000, 1.000000000000000000 ) ) ;
#14462=LINE ( 'NONE', #8334, #7370 ) ;
#14477=PLANE ( 'NONE',  #5808 ) ;
#14481=ORIENTED_EDGE ( 'NONE', *, *, #13427, .F. ) ;
#14482=CARTESIAN_POINT ( 'NONE',  ( 11.91154273188008084, 0.000000000000000000, 56.63139720814412925 ) ) ;
#14486=ADVANCED_FACE ( 'NONE', ( #7887 ), #5289, .F. ) ;
#14514=DIRECTION ( 'NONE',  ( -0.000000000000000000, -1.000000000000000000, -0.000000000000000000 ) ) ;
#14580=CARTESIAN_POINT ( 'NONE',  ( 4.896370289192182312, -3.000000000000000000, -48.48076211352908871 ) ) ;
#14581=LINE ( 'NONE', #10797, #13978 ) ;
#14590=DIRECTION ( 'NONE',  ( 0.000000000000000000, 0.000000000000000000, 1.000000000000000000 ) ) ;
#14595=ORIENTED_EDGE ( 'NONE', *, *, #11128, .T. ) ;
#14602=CARTESIAN_POINT ( 'NONE',  ( -4.618802153517017395, -5.000000000000000000, 36.00000000000000711 ) ) ;
#14616=ORIENTED_EDGE ( 'NONE', *, *, #14817, .F. ) ;
#14626=VECTOR ( 'NONE', #10711, 1000.000000000000114 ) ;
#14642=CARTESIAN_POINT ( 'NONE',  ( -28.86751345948129455, -37.00000000000000711, 49.99999999999999289 ) ) ;
#14643=EDGE_CURVE ( 'NONE', #7289, #12753, #6994, .T. ) ;
#14645=VECTOR ( 'NONE', #6344, 1000.000000000000000 ) ;
#14648=VECTOR ( 'NONE', #2107, 1000.000000000000000 ) ;
#14657=ORIENTED_EDGE ( 'NONE', *, *, #15794, .T. ) ;
#14659=ORIENTED_EDGE ( 'NONE', *, *, #13235, .F. ) ;
#14661=ORIENTED_EDGE ( 'NONE', *, *, #10397, .T. ) ;
#14663=LINE ( 'NONE', #14741, #7363 ) ;
#14679=AXIS2_PLACEMENT_3D ( 'NONE', #7424, #4091, #5067 ) ;
#14680=EDGE_LOOP ( 'NONE', ( #4659, #1039, #8300, #10921, #5319 ) ) ;
#14683=ORIENTED_EDGE ( 'NONE', *, *, #3307, .T. ) ;
#14692=VECTOR ( 'NONE', #11489, 1000.000000000000000 ) ;
#14713=CARTESIAN_POINT ( 'NONE',  ( 31.75426480542940766, -4.999999999999997335, 15.00000000000001243 ) ) ;
#14714=EDGE_CURVE ( 'NONE', #6319, #362, #10555, .T. ) ;
#14741=CARTESIAN_POINT ( 'NONE',  ( 12.67949192431120586, -37.00000000000000711, 61.96152422706632024 ) ) ;
#14760=MANIFOLD_SOLID_BREP ( 'M5 Clearance Hole1', #10510 ) ;
#14769=DIRECTION ( 'NONE',  ( -0.8660254037844387076, 0.000000000000000000, 0.4999999999999997224 ) ) ;
#14772=VERTEX_POINT ( 'NONE', #2742 ) ;
#14778=LINE ( 'NONE', #8571, #5045 ) ;
#14792=CARTESIAN_POINT ( 'NONE',  ( 30.02221399786053979, 0.000000000000000000, -15.99999999999998579 ) ) ;
#14812=DIRECTION ( 'NONE',  ( 0.8660254037844383745, 0.000000000000000000, 0.5000000000000006661 ) ) ;
#14817=EDGE_CURVE ( 'NONE', #8388, #8643, #3485, .T. ) ;
#14837=ORIENTED_EDGE ( 'NONE', *, *, #14714, .T. ) ;
#14843=AXIS2_PLACEMENT_3D ( 'NONE', #4078, #6758, #5381 ) ;
#14846=LINE ( 'NONE', #4666, #10195 ) ;
#14863=LINE ( 'NONE', #1600, #15914 ) ;
#14881=( GEOMETRIC_REPRESENTATION_CONTEXT ( 3 ) GLOBAL_UNCERTAINTY_ASSIGNED_CONTEXT ( ( #14994 ) ) GLOBAL_UNIT_ASSIGNED_CONTEXT ( ( #1475, #10128, #200 ) ) REPRESENTATION_CONTEXT ( 'NONE', 'WORKASPACE' ) );
#14890=CARTESIAN_POINT ( 'NONE',  ( 39.84679848243397515, -3.763931520638774675, 28.17238874121806091 ) ) ;
#14897=EDGE_CURVE ( 'NONE', #12880, #9400, #11783, .T. ) ;
#14898=CARTESIAN_POINT ( 'NONE',  ( 27.50000000000003197, -5.000000000000000000, -47.63139720814412925 ) ) ;
#14913=FACE_OUTER_BOUND ( 'NONE', #1784, .T. ) ;
#14940=CIRCLE ( 'NONE', #15716, 5.000000000000000000 ) ;
#14943=VECTOR ( 'NONE', #2094, 1000.000000000000000 ) ;
#14946=ORIENTED_EDGE ( 'NONE', *, *, #3783, .T. ) ;
#14950=AXIS2_PLACEMENT_3D ( 'NONE', #3671, #2531, #8384 ) ;
#14962=DIRECTION ( 'NONE',  ( 0.000000000000000000, -0.000000000000000000, 1.000000000000000000 ) ) ;
#14972=DIRECTION ( 'NONE',  ( -0.8660254037844383745, 0.000000000000000000, -0.5000000000000004441 ) ) ;
#14973=ORIENTED_EDGE ( 'NONE', *, *, #2365, .F. ) ;
#14976=EDGE_CURVE ( 'NONE', #2457, #9104, #1157, .T. ) ;
#14993=DIRECTION ( 'NONE',  ( -0.5000000000000002220, 0.000000000000000000, 0.8660254037844385966 ) ) ;
#14994=UNCERTAINTY_MEASURE_WITH_UNIT (LENGTH_MEASURE( 1.000000000000000082E-05 ), #1475, 'distance_accuracy_value', 'NONE');
#15002=CARTESIAN_POINT ( 'NONE',  ( -28.86751345948130165, 0.000000000000000000, 18.00000000000000355 ) ) ;
#15009=CARTESIAN_POINT ( 'NONE',  ( -2.886751345948099789, -37.00000000000000711, -35.00000000000000000 ) ) ;
#15050=EDGE_CURVE ( 'NONE', #15563, #15506, #14462, .T. ) ;
#15053=CIRCLE ( 'NONE', #3675, 32.00000000000000711 ) ;
#15076=ORIENTED_EDGE ( 'NONE', *, *, #15956, .T. ) ;
#15079=ORIENTED_EDGE ( 'NONE', *, *, #11261, .F. ) ;
#15089=CARTESIAN_POINT ( 'NONE',  ( -28.86751345947056180, -5.000000000000000000, -20.00000000000000355 ) ) ;
#15092=VERTEX_POINT ( 'NONE', #15601 ) ;
#15102=EDGE_LOOP ( 'NONE', ( #2290, #1252 ) ) ;
#15104=FACE_OUTER_BOUND ( 'NONE', #15944, .T. ) ;
#15106=DIRECTION ( 'NONE',  ( -0.000000000000000000, -1.000000000000000000, -0.000000000000000000 ) ) ;
#15108=( GEOMETRIC_REPRESENTATION_CONTEXT ( 3 ) GLOBAL_UNCERTAINTY_ASSIGNED_CONTEXT ( ( #13052 ) ) GLOBAL_UNIT_ASSIGNED_CONTEXT ( ( #5255, #3801, #8903 ) ) REPRESENTATION_CONTEXT ( 'NONE', 'WORKASPACE' ) );
#15121=AXIS2_PLACEMENT_3D ( 'NONE', #9379, #10894, #10746 ) ;
#15126=CARTESIAN_POINT ( 'NONE',  ( -21.01110699893041911, -3.000000000000001332, -36.39230484541334221 ) ) ;
#15136=CARTESIAN_POINT ( 'NONE',  ( 4.107478936458598184, -3.387975324182885828, -48.68990028668294912 ) ) ;
#15138=( NAMED_UNIT ( * ) SI_UNIT ( $, .STERADIAN. ) SOLID_ANGLE_UNIT ( ) );
#15160=ADVANCED_FACE ( 'NONE', ( #73 ), #4991, .F. ) ;
#15166=CARTESIAN_POINT ( 'NONE',  ( 10.17949192431120586, 0.000000000000000000, 57.63139720814412925 ) ) ;
#15168=DIRECTION ( 'NONE',  ( -0.4999999999999997780, 0.000000000000000000, -0.8660254037844388186 ) ) ;
#15184=ORIENTED_EDGE ( 'NONE', *, *, #11532, .F. ) ;
#15189=CARTESIAN_POINT ( 'NONE',  ( 47.32050807568875683, -37.00000000000000711, 41.96152422706633445 ) ) ;
#15202=CIRCLE ( 'NONE', #7985, 5.000000000000000000 ) ;
#15218=B_SPLINE_CURVE_WITH_KNOTS ( 'NONE', 3,
 ( #4794, #13581, #5271, #2511, #11170, #2763, #1558, #1474, #10212, #15136, #4056, #12374, #7634, #3819, #11253, #9006 ),
 .UNSPECIFIED., .F., .F.,
 ( 4, 2, 2, 2, 2, 2, 2, 4 ),
 ( 1.833078488450472941E-15, 0.0003988053453855977407, 0.0007976106907693624208, 0.001196416036153127209, 0.001595221381536891889, 0.002392832072304423418, 0.002791637417688189182, 0.003190442763071954946 ),
 .UNSPECIFIED. ) ;
#15244=ORIENTED_EDGE ( 'NONE', *, *, #11316, .T. ) ;
#15248=ORIENTED_EDGE ( 'NONE', *, *, #10175, .T. ) ;
#15255=EDGE_CURVE ( 'NONE', #1967, #6711, #1349, .T. ) ;
#15266=VERTEX_POINT ( 'NONE', #2720 ) ;
#15274=CARTESIAN_POINT ( 'NONE',  ( -28.86751345948129455, -37.00000000000000711, 20.00000000000000355 ) ) ;
#15279=CARTESIAN_POINT ( 'NONE',  ( -44.43375672972887003, -4.730053418719387004, -19.99999999999998934 ) ) ;
#15286=VERTEX_POINT ( 'NONE', #2809 ) ;
#15329=ORIENTED_EDGE ( 'NONE', *, *, #15050, .T. ) ;
#15335=DIRECTION ( 'NONE',  ( -0.000000000000000000, 1.000000000000000000, -0.000000000000000000 ) ) ;
#15340=CYLINDRICAL_SURFACE ( 'NONE', #8483, 5.000000000000001776 ) ;
#15351=CARTESIAN_POINT ( 'NONE',  ( -55.00000000000000000, 0.000000000000000000, -20.00000000000000711 ) ) ;
#15358=CARTESIAN_POINT ( 'NONE',  ( -44.36107179304985948, -3.978804951770219756, -20.27530572909197204 ) ) ;
#15369=VERTEX_POINT ( 'NONE', #9205 ) ;
#15382=MECHANICAL_DESIGN_GEOMETRIC_PRESENTATION_REPRESENTATION('',(#14079),#15108);
#15386=CIRCLE ( 'NONE', #13040, 40.00000000000000711 ) ;
#15388=VECTOR ( 'NONE', #9386, 1000.000000000000000 ) ;
#15399=ORIENTED_EDGE ( 'NONE', *, *, #8907, .F. ) ;
#15404=CARTESIAN_POINT ( 'NONE',  ( 39.53738644056090124, -5.000000000000000000, 28.48076211354432985 ) ) ;
#15408=DIRECTION ( 'NONE',  ( 0.000000000000000000, -1.000000000000000000, 0.000000000000000000 ) ) ;
#15415=VECTOR ( 'NONE', #12218, 1000.000000000000000 ) ;
#15441=CARTESIAN_POINT ( 'NONE',  ( 14.41154273188008439, 88.59290746114278647, 60.96152422706632024 ) ) ;
#15456=DIRECTION ( 'NONE',  ( -0.8660254037844383745, 0.000000000000000000, -0.5000000000000004441 ) ) ;
#15461=CARTESIAN_POINT ( 'NONE',  ( 39.90991147063509459, -3.660959011663038609, -28.10869455183395971 ) ) ;
#15462=EDGE_CURVE ( 'NONE', #11118, #8118, #5640, .T. ) ;
#15472=ADVANCED_FACE ( 'NONE', ( #5954 ), #4423, .F. ) ;
#15488=ORIENTED_EDGE ( 'NONE', *, *, #7135, .T. ) ;
#15492=CARTESIAN_POINT ( 'NONE',  ( 27.49999999999998224, -5.000000000000000000, 47.63139720814412925 ) ) ;
#15493=EDGE_CURVE ( 'NONE', #1764, #362, #2991, .T. ) ;
#15498=LINE ( 'NONE', #15571, #7939 ) ;
#15506=VERTEX_POINT ( 'NONE', #716 ) ;
#15509=ORIENTED_EDGE ( 'NONE', *, *, #5993, .F. ) ;
#15515=CARTESIAN_POINT ( 'NONE',  ( -28.86751345948126612, -37.00000000000000711, -20.00000000000000355 ) ) ;
#15518=CARTESIAN_POINT ( 'NONE',  ( 3.518113437216164652, -3.097286126993894495, 48.83433521136175415 ) ) ;
#15529=CARTESIAN_POINT ( 'NONE',  ( -60.00000000000000000, -37.00000000000000711, -20.00000000000000711 ) ) ;
#15532=EDGE_CURVE ( 'NONE', #13331, #9071, #14283, .T. ) ;
#15539=CARTESIAN_POINT ( 'NONE',  ( 2.875844205641825191, -3.000000000000000000, -48.98110827882413787 ) ) ;
#15547=CARTESIAN_POINT ( 'NONE',  ( 30.02221399786053979, 88.59290746114278647, -15.99999999999998579 ) ) ;
#15563=VERTEX_POINT ( 'NONE', #10953 ) ;
#15565=ORIENTED_EDGE ( 'NONE', *, *, #8773, .T. ) ;
#15567=ORIENTED_EDGE ( 'NONE', *, *, #2316, .F. ) ;
#15571=CARTESIAN_POINT ( 'NONE',  ( 3.164319481612644314, -3.000000000000000000, 49.48076211353313880 ) ) ;
#15583=EDGE_LOOP ( 'NONE', ( #2538, #2558, #12468, #4055, #13027 ) ) ;
#15594=LINE ( 'NONE', #4591, #5784 ) ;
#15601=CARTESIAN_POINT ( 'NONE',  ( -21.01110699893041911, 0.000000000000000000, -33.74230484541335073 ) ) ;
#15603=VERTEX_POINT ( 'NONE', #2309 ) ;
#15610=CARTESIAN_POINT ( 'NONE',  ( 40.36046224127503024, -3.194220869028281395, -27.64520767097959819 ) ) ;
#15638=CIRCLE ( 'NONE', #12265, 2.000000000000001776 ) ;
#15639=DIRECTION ( 'NONE',  ( 0.000000000000000000, -1.000000000000000000, 0.000000000000000000 ) ) ;
#15644=VERTEX_POINT ( 'NONE', #2619 ) ;
#15663=ORIENTED_EDGE ( 'NONE', *, *, #3366, .F. ) ;
#15668=FACE_OUTER_BOUND ( 'NONE', #2934, .T. ) ;
#15670=ADVANCED_FACE ( 'NONE', ( #8622 ), #13515, .F. ) ;
#15680=ORIENTED_EDGE ( 'NONE', *, *, #3581, .F. ) ;
#15683=VERTEX_POINT ( 'NONE', #4898 ) ;
#15688=DIRECTION ( 'NONE',  ( 0.000000000000000000, -1.000000000000000000, 0.000000000000000000 ) ) ;
#15690=LINE ( 'NONE', #8030, #15388 ) ;
#15692=EDGE_CURVE ( 'NONE', #2379, #5996, #7378, .T. ) ;
#15698=DIRECTION ( 'NONE',  ( 1.000000000000000000, 0.000000000000000000, 1.114413700119375779E-16 ) ) ;
#15699=CARTESIAN_POINT ( 'NONE',  ( 21.91530404932168352, -5.000000000000000000, -6.041579923254880136 ) ) ;
#15716=AXIS2_PLACEMENT_3D ( 'NONE', #10798, #10946, #7247 ) ;
#15728=ORIENTED_EDGE ( 'NONE', *, *, #991, .F. ) ;
#15737=LINE ( 'NONE', #11979, #14317 ) ;
#15738=CARTESIAN_POINT ( 'NONE',  ( 30.02221399786052913, 88.59290746114278647, 16.00000000000001066 ) ) ;
#15744=ORIENTED_EDGE ( 'NONE', *, *, #8305, .T. ) ;
#15755=CARTESIAN_POINT ( 'NONE',  ( -28.86751345948126257, -4.999999999999997335, -50.00000000000000711 ) ) ;
#15770=DIRECTION ( 'NONE',  ( 0.5000000000000003331, 0.000000000000000000, -0.8660254037844385966 ) ) ;
#15772=DIRECTION ( 'NONE',  ( 0.5000000000000002220, 0.000000000000000000, -0.8660254037844384856 ) ) ;
#15775=CARTESIAN_POINT ( 'NONE',  ( 39.69198092811959810, -4.097106062772730262, -28.32752661776758529 ) ) ;
#15794=EDGE_CURVE ( 'NONE', #12316, #15603, #7924, .T. ) ;
#15797=PRODUCT_DEFINITION ( 'UNKNOWN', '', #12039, #7563 ) ;
#15811=CARTESIAN_POINT ( 'NONE',  ( -21.01110699893060030, -3.000000000000001332, 36.39230484541324273 ) ) ;
#15815=EDGE_CURVE ( 'NONE', #15506, #12880, #1503, .T. ) ;
#15822=CARTESIAN_POINT ( 'NONE',  ( 14.41154273188008439, 0.000000000000000000, 60.96152422706632024 ) ) ;
#15826=DIRECTION ( 'NONE',  ( 0.000000000000000000, 0.000000000000000000, 1.000000000000000000 ) ) ;
#15827=CARTESIAN_POINT ( 'NONE',  ( 4.841222716689082439, -4.462727778340696005, 48.49605756500809406 ) ) ;
#15828=LINE ( 'NONE', #4748, #6434 ) ;
#15858=ORIENTED_EDGE ( 'NONE', *, *, #6006, .T. ) ;
#15859=CYLINDRICAL_SURFACE ( 'NONE', #12518, 29.99999999999999289 ) ;
#15862=ADVANCED_FACE ( 'NONE', ( #2787 ), #13268, .F. ) ;
#15871=VERTEX_POINT ( 'NONE', #10389 ) ;
#15907=CARTESIAN_POINT ( 'NONE',  ( 4.621606065640972538, -3.978804951770222420, 48.55546797644264245 ) ) ;
#15914=VECTOR ( 'NONE', #12495, 1000.000000000000000 ) ;
#15918=CARTESIAN_POINT ( 'NONE',  ( 42.02221399786069611, -3.000000000000000000, 1.040834085586084257E-13 ) ) ;
#15925=CARTESIAN_POINT ( 'NONE',  ( -2.886751345948103342, -37.00000000000000711, -35.00000000000000000 ) ) ;
#15937=FACE_OUTER_BOUND ( 'NONE', #12138, .T. ) ;
#15944=EDGE_LOOP ( 'NONE', ( #13951, #4630, #10860, #10450, #8971 ) ) ;
#15956=EDGE_CURVE ( 'NONE', #15563, #10113, #4558, .T. ) ;
#15958=PLANE ( 'NONE',  #5157 ) ;
ENDSEC;
END-ISO-10303-21;
